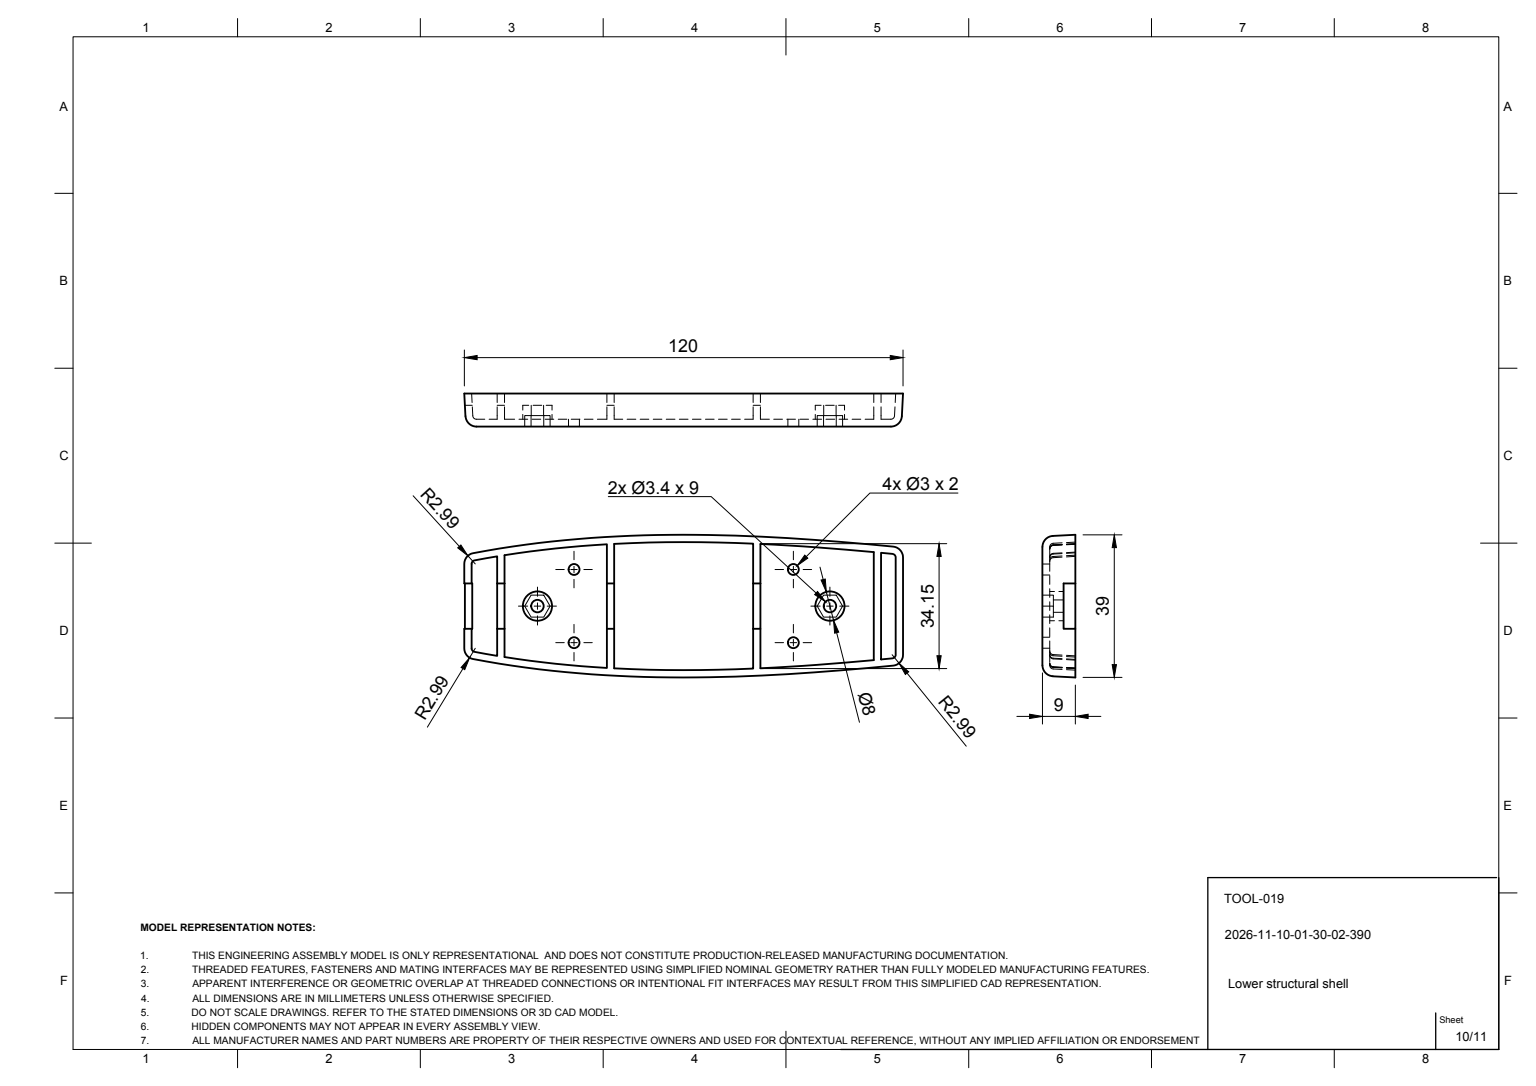
ISO-10303-21;
HEADER;
/* Generated by software containing ST-Developer
 * from STEP Tools, Inc. (www.steptools.com) 
 */

FILE_DESCRIPTION(
/* description */ (''),
/* implementation_level */ '2;1');

FILE_NAME(
/* name */ 'Lower structural shell.step',
/* time_stamp */ '2026-11-10T09:14:46-08:00',
/* author */ (''),
/* organization */ (''),
/* preprocessor_version */ 'ST-DEVELOPER v20.2',
/* originating_system */ 'Autodesk Translation Framework v15.17.0.0',
/* authorisation */ '');

FILE_SCHEMA (('AUTOMOTIVE_DESIGN { 1 0 10303 214 3 1 1 }'));
ENDSEC;

DATA;
#10=MECHANICAL_DESIGN_GEOMETRIC_PRESENTATION_REPRESENTATION('',(#563),#19471);
#84=SPHERICAL_SURFACE('',#7596,0.0999999999999999);
#85=SPHERICAL_SURFACE('',#7599,0.100000000000002);
#86=SPHERICAL_SURFACE('',#7603,0.0999999999999991);
#87=SPHERICAL_SURFACE('',#7607,0.1);
#88=SPHERICAL_SURFACE('',#7612,0.3);
#89=SPHERICAL_SURFACE('',#7616,0.300000000000002);
#90=SPHERICAL_SURFACE('',#7620,0.299999999999999);
#91=SPHERICAL_SURFACE('',#7625,0.3);
#124=B_SPLINE_SURFACE_WITH_KNOTS('',3,3,((#12681,#12682,#12683,#12684),
(#12685,#12686,#12687,#12688),(#12689,#12690,#12691,#12692),(#12693,#12694,
#12695,#12696)),.UNSPECIFIED.,.F.,.F.,.F.,(4,4),(4,4),(0.0627625298587661,
0.3242096015809),(0.0118073085896899,0.685451490706028),.UNSPECIFIED.);
#125=B_SPLINE_SURFACE_WITH_KNOTS('',3,3,((#12701,#12702,#12703,#12704),
(#12705,#12706,#12707,#12708),(#12709,#12710,#12711,#12712),(#12713,#12714,
#12715,#12716)),.UNSPECIFIED.,.F.,.F.,.F.,(4,4),(4,4),(0.0225360950145449,
0.0483865590996774),(0.0125659096559557,0.685650832343257),
 .UNSPECIFIED.);
#126=B_SPLINE_SURFACE_WITH_KNOTS('',3,3,((#12726,#12727,#12728,#12729),
(#12730,#12731,#12732,#12733),(#12734,#12735,#12736,#12737),(#12738,#12739,
#12740,#12741),(#12742,#12743,#12744,#12745)),.UNSPECIFIED.,.F.,.F.,.F.,
(4,1,4),(4,4),(0.,0.571428571428571,1.),(0.74118252158834,3.85438678954986),
 .UNSPECIFIED.);
#127=B_SPLINE_SURFACE_WITH_KNOTS('',3,3,((#12750,#12751,#12752,#12753),
(#12754,#12755,#12756,#12757),(#12758,#12759,#12760,#12761),(#12762,#12763,
#12764,#12765),(#12766,#12767,#12768,#12769)),.UNSPECIFIED.,.F.,.F.,.F.,
(4,1,4),(4,4),(0.,0.571428571428571,1.),(0.270878787657975,0.54981857912664),
 .UNSPECIFIED.);
#128=B_SPLINE_SURFACE_WITH_KNOTS('',3,3,((#12788,#12789,#12790,#12791),
(#12792,#12793,#12794,#12795),(#12796,#12797,#12798,#12799),(#12800,#12801,
#12802,#12803),(#12804,#12805,#12806,#12807)),.UNSPECIFIED.,.F.,.F.,.F.,
(4,1,4),(4,4),(0.,0.571428571428571,1.),(8.03948512627517,11.1526893942367),
 .UNSPECIFIED.);
#129=B_SPLINE_SURFACE_WITH_KNOTS('',3,3,((#12812,#12813,#12814,#12815),
(#12816,#12817,#12818,#12819),(#12820,#12821,#12822,#12823),(#12824,#12825,
#12826,#12827)),.UNSPECIFIED.,.F.,.F.,.F.,(4,4),(4,4),(0.675790398419059,
0.937237470141233),(0.0118073085603101,0.685451490706029),.UNSPECIFIED.);
#130=B_SPLINE_SURFACE_WITH_KNOTS('',3,3,((#12828,#12829,#12830,#12831),
(#12832,#12833,#12834,#12835),(#12836,#12837,#12838,#12839),(#12840,#12841,
#12842,#12843)),.UNSPECIFIED.,.F.,.F.,.F.,(4,4),(4,4),(0.951613440900322,
0.977463904985455),(0.0125659096559558,0.685650832343257),.UNSPECIFIED.);
#131=B_SPLINE_SURFACE_WITH_KNOTS('',3,3,((#12927,#12928,#12929,#12930),
(#12931,#12932,#12933,#12934),(#12935,#12936,#12937,#12938),(#12939,#12940,
#12941,#12942)),.UNSPECIFIED.,.F.,.F.,.F.,(4,4),(4,4),(0.340089900275858,
0.660082688299826),(0.0116294244283504,0.684384408933581),.UNSPECIFIED.);
#132=B_SPLINE_SURFACE_WITH_KNOTS('',3,3,((#12947,#12948,#12949,#12950),
(#12951,#12952,#12953,#12954),(#12955,#12956,#12957,#12958),(#12959,#12960,
#12961,#12962),(#12963,#12964,#12965,#12966)),.UNSPECIFIED.,.F.,.F.,.F.,
(4,1,4),(4,4),(0.,0.571428571428571,1.),(4.04989375377528,7.85140214144331),
 .UNSPECIFIED.);
#133=B_SPLINE_SURFACE_WITH_KNOTS('',3,3,((#12976,#12977,#12978,#12979),
(#12980,#12981,#12982,#12983),(#12984,#12985,#12986,#12987),(#12988,#12989,
#12990,#12991),(#12992,#12993,#12994,#12995)),.UNSPECIFIED.,.F.,.F.,.F.,
(4,1,4),(4,4),(0.,0.571428571428571,1.),(4.0424697743818,7.84397816204974),
 .UNSPECIFIED.);
#134=B_SPLINE_SURFACE_WITH_KNOTS('',3,3,((#13000,#13001,#13002,#13003),
(#13004,#13005,#13006,#13007),(#13008,#13009,#13010,#13011),(#13012,#13013,
#13014,#13015)),.UNSPECIFIED.,.F.,.F.,.F.,(4,4),(4,4),(0.339917311700174,
0.659910099724142),(0.0116294573698948,0.684384408933581),.UNSPECIFIED.);
#135=B_SPLINE_SURFACE_WITH_KNOTS('',3,3,((#13090,#13091,#13092,#13093),
(#13094,#13095,#13096,#13097),(#13098,#13099,#13100,#13101),(#13102,#13103,
#13104,#13105)),.UNSPECIFIED.,.F.,.F.,.F.,(4,4),(4,4),(0.675996615945502,
0.913173856075534),(0.0118505108223707,0.686152089762332),.UNSPECIFIED.);
#136=B_SPLINE_SURFACE_WITH_KNOTS('',3,3,((#13110,#13111,#13112,#13113),
(#13114,#13115,#13116,#13117),(#13118,#13119,#13120,#13121),(#13122,#13123,
#13124,#13125),(#13126,#13127,#13128,#13129)),.UNSPECIFIED.,.F.,.F.,.F.,
(4,1,4),(4,4),(0.,0.571428571428571,1.),(8.0457708503995,10.8690635835914),
 .UNSPECIFIED.);
#137=B_SPLINE_SURFACE_WITH_KNOTS('',3,3,((#13139,#13140,#13141,#13142),
(#13143,#13144,#13145,#13146),(#13147,#13148,#13149,#13150),(#13151,#13152,
#13153,#13154),(#13155,#13156,#13157,#13158)),.UNSPECIFIED.,.F.,.F.,.F.,
(4,1,4),(4,4),(0.,0.571428571428571,1.),(1.02480833223363,3.8481010654256),
 .UNSPECIFIED.);
#138=B_SPLINE_SURFACE_WITH_KNOTS('',3,3,((#13163,#13164,#13165,#13166),
(#13167,#13168,#13169,#13170),(#13171,#13172,#13173,#13174),(#13175,#13176,
#13177,#13178)),.UNSPECIFIED.,.F.,.F.,.F.,(4,4),(4,4),(0.0868261439244655,
0.324003384054498),(0.0118505108223707,0.686152089762332),.UNSPECIFIED.);
#139=B_SPLINE_SURFACE_WITH_KNOTS('',3,3,((#13253,#13254,#13255,#13256),
(#13257,#13258,#13259,#13260),(#13261,#13262,#13263,#13264),(#13265,#13266,
#13267,#13268)),.UNSPECIFIED.,.F.,.F.,.F.,(4,4),(4,4),(0.927751606342899,
0.979699913047832),(0.0130895688562318,0.686930956013783),.UNSPECIFIED.);
#140=B_SPLINE_SURFACE_WITH_KNOTS('',3,3,((#13278,#13279,#13280,#13281),
(#13282,#13283,#13284,#13285),(#13286,#13287,#13288,#13289),(#13290,#13291,
#13292,#13293),(#13294,#13295,#13296,#13297)),.UNSPECIFIED.,.F.,.F.,.F.,
(4,1,4),(4,4),(0.,0.571428571428571,1.),(11.0550486447215,11.6488871259622),
 .UNSPECIFIED.);
#141=B_SPLINE_SURFACE_WITH_KNOTS('',3,3,((#13311,#13312,#13313,#13314),
(#13315,#13316,#13317,#13318),(#13319,#13320,#13321,#13322),(#13323,#13324,
#13325,#13326)),.UNSPECIFIED.,.F.,.F.,.F.,(4,4),(4,4),(0.0203000869521683,
0.0722483936571013),(0.0130895688562318,0.686930956013783),
 .UNSPECIFIED.);
#142=B_SPLINE_SURFACE_WITH_KNOTS('',3,3,((#13336,#13337,#13338,#13339),
(#13340,#13341,#13342,#13343),(#13344,#13345,#13346,#13347),(#13348,#13349,
#13350,#13351),(#13352,#13353,#13354,#13355)),.UNSPECIFIED.,.F.,.F.,.F.,
(4,1,4),(4,4),(0.,0.571428571428571,1.),(0.244984789862841,0.838823271103535),
 .UNSPECIFIED.);
#143=B_SPLINE_SURFACE_WITH_KNOTS('',3,3,((#13369,#13370,#13371,#13372),
(#13373,#13374,#13375,#13376),(#13377,#13378,#13379,#13380),(#13381,#13382,
#13383,#13384),(#13385,#13386,#13387,#13388)),.UNSPECIFIED.,.F.,.F.,.F.,
(4,1,4),(4,4),(0.,0.5,1.),(0.0108921325678979,0.619909717328002),
 .UNSPECIFIED.);
#144=B_SPLINE_SURFACE_WITH_KNOTS('',3,3,((#13395,#13396,#13397,#13398),
(#13399,#13400,#13401,#13402),(#13403,#13404,#13405,#13406),(#13407,#13408,
#13409,#13410),(#13411,#13412,#13413,#13414)),.UNSPECIFIED.,.F.,.F.,.F.,
(4,1,4),(4,4),(0.,0.571428571428571,1.),(0.00967450486392679,0.618764321025346),
 .UNSPECIFIED.);
#145=B_SPLINE_SURFACE_WITH_KNOTS('',3,3,((#13419,#13420,#13421,#13422),
(#13423,#13424,#13425,#13426),(#13427,#13428,#13429,#13430),(#13431,#13432,
#13433,#13434),(#13435,#13436,#13437,#13438)),.UNSPECIFIED.,.F.,.F.,.F.,
(4,1,4),(4,4),(0.,0.571428571428571,1.),(0.0097274579809394,0.618764321025346),
 .UNSPECIFIED.);
#146=B_SPLINE_SURFACE_WITH_KNOTS('',3,3,((#13443,#13444,#13445,#13446),
(#13447,#13448,#13449,#13450),(#13451,#13452,#13453,#13454),(#13455,#13456,
#13457,#13458),(#13459,#13460,#13461,#13462)),.UNSPECIFIED.,.F.,.F.,.F.,
(4,1,4),(4,4),(0.,0.571428571428571,1.),(11.3440533366984,11.6229931281671),
 .UNSPECIFIED.);
#147=B_SPLINE_SURFACE_WITH_KNOTS('',3,3,((#13463,#13464,#13465,#13466),
(#13467,#13468,#13469,#13470),(#13471,#13472,#13473,#13474),(#13475,#13476,
#13477,#13478),(#13479,#13480,#13481,#13482)),.UNSPECIFIED.,.F.,.F.,.F.,
(4,1,4),(4,4),(0.,0.5,1.),(0.0108402259132964,0.619909717328002),
 .UNSPECIFIED.);
#148=B_SPLINE_SURFACE_WITH_KNOTS('',3,3,((#13508,#13509,#13510,#13511),
(#13512,#13513,#13514,#13515),(#13516,#13517,#13518,#13519),(#13520,#13521,
#13522,#13523),(#13524,#13525,#13526,#13527)),.UNSPECIFIED.,.F.,.F.,.F.,
(4,1,4),(4,4),(0.,0.571428571428571,1.),(-0.00387706229521417,0.619909717328002),
 .UNSPECIFIED.);
#149=B_SPLINE_SURFACE_WITH_KNOTS('',3,3,((#13546,#13547,#13548,#13549,#13550,
#13551),(#13552,#13553,#13554,#13555,#13556,#13557),(#13558,#13559,#13560,
#13561,#13562,#13563),(#13564,#13565,#13566,#13567,#13568,#13569),(#13570,
#13571,#13572,#13573,#13574,#13575)),.UNSPECIFIED.,.F.,.F.,.F.,(4,1,4),
(4,1,1,4),(0.,0.571428571428571,1.),(0.270878787657975,5.14716807550265,
8.39802760073243,11.6488871259622),.UNSPECIFIED.);
#150=B_SPLINE_SURFACE_WITH_KNOTS('',3,3,((#13588,#13589,#13590,#13591),
(#13592,#13593,#13594,#13595),(#13596,#13597,#13598,#13599),(#13600,#13601,
#13602,#13603),(#13604,#13605,#13606,#13607)),.UNSPECIFIED.,.F.,.F.,.F.,
(4,1,4),(4,4),(0.,0.571428571428571,1.),(-0.00522825793187074,0.618764321025346),
 .UNSPECIFIED.);
#151=B_SPLINE_SURFACE_WITH_KNOTS('',3,3,((#13616,#13617,#13618,#13619),
(#13620,#13621,#13622,#13623),(#13624,#13625,#13626,#13627),(#13628,#13629,
#13630,#13631),(#13632,#13633,#13634,#13635)),.UNSPECIFIED.,.F.,.F.,.F.,
(4,1,4),(4,4),(0.,0.571428571428571,1.),(-0.00506942997988007,0.618764321025346),
 .UNSPECIFIED.);
#152=B_SPLINE_SURFACE_WITH_KNOTS('',3,3,((#13644,#13645,#13646,#13647,#13648),
(#13649,#13650,#13651,#13652,#13653),(#13654,#13655,#13656,#13657,#13658),
(#13659,#13660,#13661,#13662,#13663),(#13664,#13665,#13666,#13667,#13668)),
 .UNSPECIFIED.,.F.,.F.,.F.,(4,1,4),(4,1,4),(0.,0.571428571428571,1.),(0.244984789862841,
5.12127407770751,11.6229931281671),.UNSPECIFIED.);
#153=B_SPLINE_SURFACE_WITH_KNOTS('',3,3,((#13679,#13680,#13681,#13682),
(#13683,#13684,#13685,#13686),(#13687,#13688,#13689,#13690),(#13691,#13692,
#13693,#13694),(#13695,#13696,#13697,#13698)),.UNSPECIFIED.,.F.,.F.,.F.,
(4,1,4),(4,4),(0.,0.571428571428571,1.),(-0.00403278922781227,0.619909717328002),
 .UNSPECIFIED.);
#154=B_SPLINE_SURFACE_WITH_KNOTS('',3,3,((#13707,#13708,#13709,#13710),
(#13711,#13712,#13713,#13714),(#13715,#13716,#13717,#13718),(#13719,#13720,
#13721,#13722)),.UNSPECIFIED.,.F.,.F.,.F.,(4,4),(4,4),(0.0225340877622934,
0.979701609653785),(0.,0.686930956013783),.UNSPECIFIED.);
#155=B_SPLINE_SURFACE_WITH_KNOTS('',3,3,((#13725,#13726,#13727,#13728),
(#13729,#13730,#13731,#13732),(#13733,#13734,#13735,#13736),(#13737,#13738,
#13739,#13740)),.UNSPECIFIED.,.F.,.F.,.F.,(4,4),(4,4),(0.0202983903462145,
0.977465912237707),(0.,0.686930956013783),.UNSPECIFIED.);
#264=B_SPLINE_CURVE_WITH_KNOTS('',3,(#11953,#11954,#11955,#11956,#11957,
#11958),.UNSPECIFIED.,.F.,.F.,(4,2,4),(-0.607240122656937,-0.303691721894415,
-0.000634514333697656),.UNSPECIFIED.);
#265=B_SPLINE_CURVE_WITH_KNOTS('',3,(#11960,#11961,#11962,#11963,#11964,
#11965,#11966,#11967,#11968,#11969,#11970,#11971,#11972,#11973,#11974,#11975,
#11976,#11977,#11978,#11979,#11980,#11981,#11982,#11983,#11984,#11985,#11986,
#11987),.UNSPECIFIED.,.F.,.F.,(4,3,3,3,3,3,3,3,3,4),(-0.152223584381152,
-0.128403685910756,-0.115058138924018,-0.0911105876986024,-0.0779275105489685,
-0.0651650823668383,-0.0413494676927402,-0.0389105926748606,-0.0151313403168948,
0.),.UNSPECIFIED.);
#266=B_SPLINE_CURVE_WITH_KNOTS('',3,(#11991,#11992,#11993,#11994,#11995,
#11996,#11997,#11998,#11999,#12000,#12001,#12002,#12003,#12004,#12005,#12006,
#12007,#12008,#12009,#12010,#12011,#12012,#12013,#12014,#12015,#12016,#12017,
#12018),.UNSPECIFIED.,.F.,.F.,(4,3,3,3,3,3,3,3,3,4),(-0.152249917238265,
-0.128484865669312,-0.115494642307313,-0.0916985948709881,-0.0870953287403626,
-0.0787006597758974,-0.0547717013112817,-0.0393956522318865,-0.0155460991587222,
0.),.UNSPECIFIED.);
#267=B_SPLINE_CURVE_WITH_KNOTS('',3,(#12019,#12020,#12021,#12022,#12023,
#12024),.UNSPECIFIED.,.F.,.F.,(4,2,4),(-0.606785315485727,-0.30369188913634,
-0.000179692314978108),.UNSPECIFIED.);
#268=B_SPLINE_CURVE_WITH_KNOTS('',3,(#12029,#12030,#12031,#12032,#12033,
#12034),.UNSPECIFIED.,.F.,.F.,(4,2,4),(-0.606332812995025,-0.303737653350621,
-0.000161665236032726),.UNSPECIFIED.);
#269=B_SPLINE_CURVE_WITH_KNOTS('',3,(#12036,#12037,#12038,#12039,#12040,
#12041,#12042,#12043,#12044,#12045,#12046,#12047,#12048,#12049,#12050,#12051,
#12052,#12053,#12054,#12055,#12056,#12057,#12058,#12059,#12060,#12061,#12062,
#12063),.UNSPECIFIED.,.F.,.F.,(4,3,3,3,3,3,3,3,3,4),(-0.152301160038588,
-0.128555435257278,-0.115184785848022,-0.0912639339035621,-0.0780773216554274,
-0.065267350293706,-0.0414723266145325,-0.0390252168402571,-0.0152374671294611,
0.),.UNSPECIFIED.);
#270=B_SPLINE_CURVE_WITH_KNOTS('',3,(#12067,#12068,#12069,#12070,#12071,
#12072,#12073,#12074,#12075,#12076,#12077,#12078,#12079,#12080,#12081,#12082,
#12083,#12084,#12085,#12086,#12087,#12088,#12089,#12090,#12091,#12092,#12093,
#12094),.UNSPECIFIED.,.F.,.F.,(4,3,3,3,3,3,3,3,3,4),(-0.152307894271445,
-0.128535938708366,-0.115295945509717,-0.0915234088298753,-0.0870575315710991,
-0.0782740392368046,-0.0543664511067997,-0.0391484926712317,-0.0153774171089249,
0.),.UNSPECIFIED.);
#271=B_SPLINE_CURVE_WITH_KNOTS('',3,(#12096,#12097,#12098,#12099,#12100,
#12101),.UNSPECIFIED.,.F.,.F.,(4,2,4),(-0.607315067615316,-0.303737782617996,
-0.00114390098251854),.UNSPECIFIED.);
#272=B_SPLINE_CURVE_WITH_KNOTS('',3,(#12107,#12108,#12109,#12110,#12111,
#12112),.UNSPECIFIED.,.F.,.F.,(4,2,4),(-0.606335618682527,-0.303964064424246,
-0.000163142902895597),.UNSPECIFIED.);
#273=B_SPLINE_CURVE_WITH_KNOTS('',3,(#12114,#12115,#12116,#12117,#12118,
#12119,#12120,#12121,#12122,#12123,#12124,#12125,#12126,#12127,#12128,#12129,
#12130,#12131,#12132,#12133,#12134,#12135,#12136,#12137,#12138,#12139,#12140,
#12141),.UNSPECIFIED.,.F.,.F.,(4,3,3,3,3,3,3,3,3,4),(-0.152324888062519,
-0.128571266282871,-0.115187819092559,-0.0912644922975459,-0.0780623053857969,
-0.0652705430018984,-0.0414736125245103,-0.0390138150290758,-0.015226502089553,
0.),.UNSPECIFIED.);
#274=B_SPLINE_CURVE_WITH_KNOTS('',3,(#12145,#12146,#12147,#12148,#12149,
#12150,#12151,#12152,#12153,#12154,#12155,#12156,#12157,#12158,#12159,#12160,
#12161,#12162,#12163,#12164,#12165,#12166,#12167,#12168,#12169,#12170,#12171,
#12172),.UNSPECIFIED.,.F.,.F.,(4,3,3,3,3,3,3,3,3,4),(-0.152333600285603,
-0.128561769460285,-0.115331525958272,-0.0915566852459163,-0.0870792380259527,
-0.0783165909319309,-0.0544069520497563,-0.0391732033593778,-0.0153939862842036,
0.),.UNSPECIFIED.);
#275=B_SPLINE_CURVE_WITH_KNOTS('',3,(#12174,#12175,#12176,#12177,#12178,
#12179),.UNSPECIFIED.,.F.,.F.,(4,2,4),(-0.607765665607205,-0.303964210965506,
-0.00159316434717749),.UNSPECIFIED.);
#276=B_SPLINE_CURVE_WITH_KNOTS('',3,(#12185,#12186,#12187,#12188,#12189,
#12190),.UNSPECIFIED.,.F.,.F.,(4,2,4),(-0.608113833554089,-0.304405910662044,
-0.00120843896277512),.UNSPECIFIED.);
#277=B_SPLINE_CURVE_WITH_KNOTS('',3,(#12192,#12193,#12194,#12195,#12196,
#12197,#12198,#12199,#12200,#12201,#12202,#12203,#12204,#12205,#12206,#12207,
#12208,#12209,#12210,#12211,#12212,#12213,#12214,#12215,#12216,#12217,#12218,
#12219),.UNSPECIFIED.,.F.,.F.,(4,3,3,3,3,3,3,3,3,4),(-0.152638346832965,
-0.128647829044501,-0.117000727359648,-0.0929750760194364,-0.0775532335837778,
-0.065166230851578,-0.0413072760700971,-0.0386249916896363,-0.0148681833632798,
0.),.UNSPECIFIED.);
#278=B_SPLINE_CURVE_WITH_KNOTS('',3,(#12223,#12224,#12225,#12226,#12227,
#12228,#12229,#12230,#12231,#12232,#12233,#12234,#12235,#12236,#12237,#12238,
#12239,#12240,#12241,#12242,#12243,#12244,#12245,#12246,#12247,#12248,#12249,
#12250),.UNSPECIFIED.,.F.,.F.,(4,3,3,3,3,3,3,3,3,4),(-0.152712908768378,
-0.128963682254188,-0.116304008925778,-0.092453135123643,-0.0875380734791113,
-0.0797852913889514,-0.0558105568475602,-0.0400274901149945,-0.0159798645019078,
0.),.UNSPECIFIED.);
#279=B_SPLINE_CURVE_WITH_KNOTS('',3,(#12252,#12253,#12254,#12255,#12256,
#12257),.UNSPECIFIED.,.F.,.F.,(4,2,4),(-0.607607610897069,-0.304406883675693,
-0.000702187548907163),.UNSPECIFIED.);
#280=B_SPLINE_CURVE_WITH_KNOTS('',3,(#12263,#12264,#12265,#12266),
 .UNSPECIFIED.,.F.,.F.,(4,4),(0.0130288733793136,0.619909717328002),
 .UNSPECIFIED.);
#281=B_SPLINE_CURVE_WITH_KNOTS('',3,(#12270,#12271,#12272,#12273),
 .UNSPECIFIED.,.F.,.F.,(4,4),(-0.619909717328002,-0.0130288733793137),
 .UNSPECIFIED.);
#282=B_SPLINE_CURVE_WITH_KNOTS('',3,(#12276,#12277,#12278,#12279,#12280,
#12281,#12282),.UNSPECIFIED.,.F.,.F.,(4,3,4),(7.87274532319472,10.4298004347969,
10.9780233963721),.UNSPECIFIED.);
#283=B_SPLINE_CURVE_WITH_KNOTS('',3,(#12283,#12284,#12285,#12286,#12287,
#12288,#12289),.UNSPECIFIED.,.F.,.F.,(4,3,4),(0.511752108249611,2.84807862798167,
3.61537599721027),.UNSPECIFIED.);
#284=B_SPLINE_CURVE_WITH_KNOTS('',3,(#12292,#12293,#12294,#12295,#12296,
#12297,#12298),.UNSPECIFIED.,.F.,.F.,(4,3,4),(3.81523717927831,5.72635044542746,
7.61820606472736),.UNSPECIFIED.);
#285=B_SPLINE_CURVE_WITH_KNOTS('',3,(#12301,#12302,#12303,#12304),
 .UNSPECIFIED.,.F.,.F.,(4,4),(7.8195516254834,10.6519234170402),
 .UNSPECIFIED.);
#286=B_SPLINE_CURVE_WITH_KNOTS('',3,(#12308,#12309,#12310,#12311),
 .UNSPECIFIED.,.F.,.F.,(4,4),(10.8550709503701,11.4839159448819),
 .UNSPECIFIED.);
#287=B_SPLINE_CURVE_WITH_KNOTS('',3,(#12312,#12313,#12314,#12315,#12316,
#12317,#12318,#12319,#12320,#12321,#12322,#12323,#12324,#12325,#12326,#12327,
#12328,#12329,#12330,#12331,#12332,#12333,#12334,#12335,#12336,#12337,#12338,
#12339),.UNSPECIFIED.,.F.,.F.,(4,3,3,3,3,3,3,3,3,4),(0.,0.023800266251022,
0.0390470051780055,0.062864594207143,0.0692752090304052,0.0780196763370091,
0.101808338076191,0.108235461704482,0.131970324379069,0.138468980573541),
 .UNSPECIFIED.);
#288=B_SPLINE_CURVE_WITH_KNOTS('',3,(#12343,#12344,#12345,#12346,#12347,
#12348,#12349,#12350,#12351,#12352,#12353,#12354,#12355,#12356,#12357,#12358,
#12359,#12360,#12361,#12362,#12363,#12364,#12365,#12366,#12367,#12368,#12369,
#12370,#12371,#12372,#12373),.UNSPECIFIED.,.F.,.F.,(4,3,3,3,3,3,3,3,3,3,
4),(0.,0.0536158767337707,0.107707970980176,0.117140678528723,0.171373940961503,
0.178118425384842,0.234058785038521,0.2884659822146,0.324708667187819,0.378759781373182,
0.415412568437851),.UNSPECIFIED.);
#289=B_SPLINE_CURVE_WITH_KNOTS('',3,(#12375,#12376,#12377,#12378),
 .UNSPECIFIED.,.F.,.F.,(4,4),(0.0202983903462145,0.977465912237707),
 .UNSPECIFIED.);
#290=B_SPLINE_CURVE_WITH_KNOTS('',3,(#12380,#12381,#12382,#12383,#12384,
#12385,#12386,#12387,#12388,#12389,#12390,#12391,#12392,#12393,#12394,#12395,
#12396,#12397,#12398,#12399,#12400,#12401,#12402,#12403,#12404,#12405,#12406,
#12407,#12408,#12409,#12410),.UNSPECIFIED.,.F.,.F.,(4,3,3,3,3,3,3,3,3,3,
4),(0.,0.053547205187505,0.107728964525782,0.117299670245694,0.171524652009909,
0.189842726242433,0.234296321023441,0.288773621215207,0.338477936388461,
0.392564001789548,0.442713223041249),.UNSPECIFIED.);
#291=B_SPLINE_CURVE_WITH_KNOTS('',3,(#12414,#12415,#12416,#12417,#12418,
#12419,#12420,#12421,#12422,#12423,#12424,#12425,#12426,#12427,#12428,#12429,
#12430,#12431,#12432,#12433,#12434,#12435,#12436,#12437,#12438,#12439,#12440,
#12441,#12442,#12443,#12444),.UNSPECIFIED.,.F.,.F.,(4,3,3,3,3,3,3,3,3,3,
4),(0.,0.0535312152416108,0.107707123412492,0.117215931328448,0.171445047002381,
0.189808362521926,0.234165405003858,0.288639615809812,0.338404447092272,
0.392504428396833,0.442708851597914),.UNSPECIFIED.);
#292=B_SPLINE_CURVE_WITH_KNOTS('',3,(#12446,#12447,#12448,#12449),
 .UNSPECIFIED.,.F.,.F.,(4,4),(0.0225340877622936,0.979701609653785),
 .UNSPECIFIED.);
#293=B_SPLINE_CURVE_WITH_KNOTS('',3,(#12451,#12452,#12453,#12454,#12455,
#12456,#12457,#12458,#12459,#12460,#12461,#12462,#12463,#12464,#12465,#12466,
#12467,#12468,#12469,#12470,#12471,#12472,#12473,#12474,#12475,#12476,#12477,
#12478,#12479,#12480,#12481),.UNSPECIFIED.,.F.,.F.,(4,3,3,3,3,3,3,3,3,3,
4),(0.,0.0536458552170769,0.107744721567334,0.117297895480617,0.171522683869793,
0.178177673384308,0.23429412186666,0.288702228477357,0.324838815929715,
0.378862861687027,0.415420074045746),.UNSPECIFIED.);
#294=B_SPLINE_CURVE_WITH_KNOTS('',3,(#12484,#12485,#12486,#12487,#12488,
#12489,#12490,#12491,#12492,#12493,#12494,#12495,#12496,#12497,#12498,#12499,
#12500,#12501,#12502,#12503,#12504,#12505,#12506,#12507,#12508,#12509,#12510,
#12511),.UNSPECIFIED.,.F.,.F.,(4,3,3,3,3,3,3,3,3,4),(0.,0.0238098951475563,
0.0390995920428052,0.0629117710415135,0.0692953339558167,0.0780985718814299,
0.101889748471939,0.108278926258091,0.132003149848588,0.138471484390145),
 .UNSPECIFIED.);
#295=B_SPLINE_CURVE_WITH_KNOTS('',3,(#12513,#12514,#12515,#12516),
 .UNSPECIFIED.,.F.,.F.,(4,4),(2.05597917304345E-5,0.629200412657851),
 .UNSPECIFIED.);
#296=B_SPLINE_CURVE_WITH_KNOTS('',3,(#12519,#12520,#12521,#12522),
 .UNSPECIFIED.,.F.,.F.,(4,4),(0.832456091119126,3.6663340257767),
 .UNSPECIFIED.);
#297=B_SPLINE_CURVE_WITH_KNOTS('',3,(#12525,#12526,#12527,#12528,#12529,
#12530,#12531),.UNSPECIFIED.,.F.,.F.,(4,3,4),(3.86778652923942,5.76006783397632,
7.67277763234621),.UNSPECIFIED.);
#298=B_SPLINE_CURVE_WITH_KNOTS('',3,(#12535,#12536,#12537,#12538),
 .UNSPECIFIED.,.F.,.F.,(4,4),(11.1789026308149,11.490024089745),
 .UNSPECIFIED.);
#299=B_SPLINE_CURVE_WITH_KNOTS('',3,(#12540,#12541,#12542,#12543,#12544,
#12545,#12546,#12547,#12548,#12549,#12550,#12551,#12552,#12553,#12554,#12555,
#12556,#12557,#12558,#12559,#12560,#12561,#12562,#12563,#12564),
 .UNSPECIFIED.,.F.,.F.,(4,3,3,3,3,3,3,3,4),(0.,0.0238050540413609,0.0390723036702896,
0.0632692088215501,0.0780555758269344,0.101951849921082,0.112801451778717,
0.136536488207902,0.147568670144067),.UNSPECIFIED.);
#300=B_SPLINE_CURVE_WITH_KNOTS('',3,(#12568,#12569,#12570,#12571,#12572,
#12573,#12574,#12575,#12576,#12577,#12578,#12579,#12580,#12581,#12582,#12583,
#12584,#12585,#12586,#12587,#12588,#12589,#12590,#12591,#12592),
 .UNSPECIFIED.,.F.,.F.,(4,3,3,3,3,3,3,3,4),(0.,0.0238098889950854,0.0391003179068551,
0.0632803937136523,0.0780994777107358,0.101997157448698,0.112825962756833,
0.136555142506291,0.147570127973408),.UNSPECIFIED.);
#301=B_SPLINE_CURVE_WITH_KNOTS('',3,(#12594,#12595,#12596,#12597),
 .UNSPECIFIED.,.F.,.F.,(4,4),(2.41556456535008E-5,0.310979882704647),
 .UNSPECIFIED.);
#302=B_SPLINE_CURVE_WITH_KNOTS('',3,(#12609,#12610,#12611,#12612,#12613,
#12614),.UNSPECIFIED.,.F.,.F.,(4,2,4),(-0.606744425054929,-0.30369469419025,
-0.000104868936493974),.UNSPECIFIED.);
#303=B_SPLINE_CURVE_WITH_KNOTS('',3,(#12616,#12617,#12618,#12619,#12620,
#12621),.UNSPECIFIED.,.F.,.F.,(4,2,4),(-0.60732337425873,-0.303694522808999,
-0.000683832228057069),.UNSPECIFIED.);
#304=B_SPLINE_CURVE_WITH_KNOTS('',3,(#12623,#12624,#12625,#12626,#12627,
#12628,#12629,#12630,#12631,#12632,#12633,#12634,#12635,#12636,#12637,#12638,
#12639,#12640,#12641,#12642,#12643,#12644,#12645,#12646,#12647,#12648,#12649,
#12650),.UNSPECIFIED.,.F.,.F.,(4,3,3,3,3,3,3,3,3,4),(-0.152213081758773,
-0.128388856548194,-0.115047734630008,-0.0910986092737131,-0.0779187269986961,
-0.0651565114518209,-0.0413397067626705,-0.0389038209724845,-0.0151251319644201,
0.),.UNSPECIFIED.);
#305=B_SPLINE_CURVE_WITH_KNOTS('',3,(#12653,#12654,#12655,#12656,#12657,
#12658,#12659,#12660,#12661,#12662,#12663,#12664,#12665,#12666,#12667,#12668,
#12669,#12670,#12671,#12672,#12673,#12674,#12675,#12676,#12677,#12678,#12679,
#12680),.UNSPECIFIED.,.F.,.F.,(4,3,3,3,3,3,3,3,3,4),(-0.152240567100014,
-0.128476012965191,-0.115503482174674,-0.0917060839439778,-0.0870941983819305,
-0.0787260045726768,-0.0547958477503903,-0.0394103419198022,-0.0155561788900784,
0.),.UNSPECIFIED.);
#306=B_SPLINE_CURVE_WITH_KNOTS('',3,(#12697,#12698,#12699,#12700),
 .UNSPECIFIED.,.F.,.F.,(4,4),(-3.85438678954986,-0.750511952447855),
 .UNSPECIFIED.);
#307=B_SPLINE_CURVE_WITH_KNOTS('',3,(#12718,#12719,#12720,#12721),
 .UNSPECIFIED.,.F.,.F.,(4,4),(-0.54981857912664,-0.270878787657975),
 .UNSPECIFIED.);
#308=B_SPLINE_CURVE_WITH_KNOTS('',3,(#12722,#12723,#12724,#12725),
 .UNSPECIFIED.,.F.,.F.,(4,4),(-0.618764321025346,-0.0114172178585034),
 .UNSPECIFIED.);
#309=B_SPLINE_CURVE_WITH_KNOTS('',3,(#12746,#12747,#12748,#12749),
 .UNSPECIFIED.,.F.,.F.,(4,4),(0.74118252158834,3.84969085360113),
 .UNSPECIFIED.);
#310=B_SPLINE_CURVE_WITH_KNOTS('',3,(#12771,#12772,#12773,#12774),
 .UNSPECIFIED.,.F.,.F.,(4,4),(0.270878787657975,0.540284107299618),
 .UNSPECIFIED.);
#311=B_SPLINE_CURVE_WITH_KNOTS('',3,(#12777,#12778,#12779,#12780),
 .UNSPECIFIED.,.F.,.F.,(4,4),(8.04418106222393,11.1526893942367),
 .UNSPECIFIED.);
#312=B_SPLINE_CURVE_WITH_KNOTS('',3,(#12783,#12784,#12785,#12786),
 .UNSPECIFIED.,.F.,.F.,(4,4),(11.3535878085254,11.6229931281671),
 .UNSPECIFIED.);
#313=B_SPLINE_CURVE_WITH_KNOTS('',3,(#12808,#12809,#12810,#12811),
 .UNSPECIFIED.,.F.,.F.,(4,4),(-11.1433599633772,-8.03948512627517),
 .UNSPECIFIED.);
#314=B_SPLINE_CURVE_WITH_KNOTS('',3,(#12845,#12846,#12847,#12848),
 .UNSPECIFIED.,.F.,.F.,(4,4),(0.0114172178585033,0.618764321025346),
 .UNSPECIFIED.);
#315=B_SPLINE_CURVE_WITH_KNOTS('',3,(#12849,#12850,#12851,#12852),
 .UNSPECIFIED.,.F.,.F.,(4,4),(-11.6229931281671,-11.3440533366984),
 .UNSPECIFIED.);
#316=B_SPLINE_CURVE_WITH_KNOTS('',3,(#12855,#12856,#12857,#12858,#12859,
#12860),.UNSPECIFIED.,.F.,.F.,(4,2,4),(-0.606286853269513,-0.303735636734938,
-0.000134370544016882),.UNSPECIFIED.);
#317=B_SPLINE_CURVE_WITH_KNOTS('',3,(#12862,#12863,#12864,#12865,#12866,
#12867,#12868,#12869,#12870,#12871,#12872,#12873,#12874,#12875,#12876,#12877,
#12878,#12879,#12880,#12881,#12882,#12883,#12884,#12885,#12886,#12887,#12888,
#12889),.UNSPECIFIED.,.F.,.F.,(4,3,3,3,3,3,3,3,3,4),(-0.152301724526365,
-0.128559761662057,-0.115189905045126,-0.0912708316251271,-0.0780855696141105,
-0.0652713768517459,-0.0414777101816728,-0.0390314967756457,-0.015242903619151,
0.),.UNSPECIFIED.);
#318=B_SPLINE_CURVE_WITH_KNOTS('',3,(#12893,#12894,#12895,#12896,#12897,
#12898,#12899,#12900,#12901,#12902,#12903,#12904,#12905,#12906,#12907,#12908,
#12909,#12910,#12911,#12912,#12913,#12914,#12915,#12916,#12917,#12918,#12919,
#12920),.UNSPECIFIED.,.F.,.F.,(4,3,3,3,3,3,3,3,3,4),(-0.1523073815286,-0.1285346644938,
-0.115283264026726,-0.0915123087981378,-0.0870533687950649,-0.0782507800682277,
-0.0543447803816484,-0.0391350231834537,-0.0153679399182895,0.),
 .UNSPECIFIED.);
#319=B_SPLINE_CURVE_WITH_KNOTS('',3,(#12921,#12922,#12923,#12924,#12925,
#12926),.UNSPECIFIED.,.F.,.F.,(4,2,4),(-0.607338074051965,-0.303735662161239,
-0.00118557149519966),.UNSPECIFIED.);
#320=B_SPLINE_CURVE_WITH_KNOTS('',3,(#12943,#12944,#12945,#12946),
 .UNSPECIFIED.,.F.,.F.,(4,4),(-7.8460657686783,-4.05419673417835),
 .UNSPECIFIED.);
#321=B_SPLINE_CURVE_WITH_KNOTS('',3,(#12967,#12968,#12969,#12970),
 .UNSPECIFIED.,.F.,.F.,(4,4),(4.04989375377528,7.85140214144331),
 .UNSPECIFIED.);
#322=B_SPLINE_CURVE_WITH_KNOTS('',3,(#12972,#12973,#12974,#12975),
 .UNSPECIFIED.,.F.,.F.,(4,4),(4.0424697743818,7.84397816204974),
 .UNSPECIFIED.);
#323=B_SPLINE_CURVE_WITH_KNOTS('',3,(#12996,#12997,#12998,#12999),
 .UNSPECIFIED.,.F.,.F.,(4,4),(-7.83967518164668,-4.0478061471468),
 .UNSPECIFIED.);
#324=B_SPLINE_CURVE_WITH_KNOTS('',3,(#13018,#13019,#13020,#13021,#13022,
#13023),.UNSPECIFIED.,.F.,.F.,(4,2,4),(-0.606398914035431,-0.303967092551845,
-0.000200694235479137),.UNSPECIFIED.);
#325=B_SPLINE_CURVE_WITH_KNOTS('',3,(#13025,#13026,#13027,#13028,#13029,
#13030,#13031,#13032,#13033,#13034,#13035,#13036,#13037,#13038,#13039,#13040,
#13041,#13042,#13043,#13044,#13045,#13046,#13047,#13048,#13049,#13050,#13051,
#13052),.UNSPECIFIED.,.F.,.F.,(4,3,3,3,3,3,3,3,3,4),(-0.15233244131821,
-0.128569871170003,-0.115181988990177,-0.0912564475476021,-0.0780459432968613,
-0.0652662335163151,-0.0414674738832469,-0.0390013640446512,-0.0152139229936509,
0.),.UNSPECIFIED.);
#326=B_SPLINE_CURVE_WITH_KNOTS('',3,(#13056,#13057,#13058,#13059,#13060,
#13061,#13062,#13063,#13064,#13065,#13066,#13067,#13068,#13069,#13070,#13071,
#13072,#13073,#13074,#13075,#13076,#13077,#13078,#13079,#13080,#13081,#13082,
#13083),.UNSPECIFIED.,.F.,.F.,(4,3,3,3,3,3,3,3,3,4),(-0.152343297533924,
-0.128571042154168,-0.115361098257144,-0.0915841820623439,-0.0870924557961151,
-0.0783628838319633,-0.0544516462338148,-0.0392000432438046,-0.0154115240971992,
0.),.UNSPECIFIED.);
#327=B_SPLINE_CURVE_WITH_KNOTS('',3,(#13084,#13085,#13086,#13087,#13088,
#13089),.UNSPECIFIED.,.F.,.F.,(4,2,4),(-0.607734321217702,-0.303967174049374,
-0.00153607519677973),.UNSPECIFIED.);
#328=B_SPLINE_CURVE_WITH_KNOTS('',3,(#13106,#13107,#13108,#13109),
 .UNSPECIFIED.,.F.,.F.,(4,4),(-10.8531956503852,-8.0457708503995),
 .UNSPECIFIED.);
#329=B_SPLINE_CURVE_WITH_KNOTS('',3,(#13130,#13131,#13132,#13133),
 .UNSPECIFIED.,.F.,.F.,(4,4),(8.05172912332209,10.8690635835914),
 .UNSPECIFIED.);
#330=B_SPLINE_CURVE_WITH_KNOTS('',3,(#13135,#13136,#13137,#13138),
 .UNSPECIFIED.,.F.,.F.,(4,4),(1.02480833223363,3.84214279250303),
 .UNSPECIFIED.);
#331=B_SPLINE_CURVE_WITH_KNOTS('',3,(#13159,#13160,#13161,#13162),
 .UNSPECIFIED.,.F.,.F.,(4,4),(-3.8481010654256,-1.04067626543981),
 .UNSPECIFIED.);
#332=B_SPLINE_CURVE_WITH_KNOTS('',3,(#13181,#13182,#13183,#13184,#13185,
#13186),.UNSPECIFIED.,.F.,.F.,(4,2,4),(-0.608301643694891,-0.304416323412316,
-0.0013178649037765),.UNSPECIFIED.);
#333=B_SPLINE_CURVE_WITH_KNOTS('',3,(#13188,#13189,#13190,#13191,#13192,
#13193,#13194,#13195,#13196,#13197,#13198,#13199,#13200,#13201,#13202,#13203,
#13204,#13205,#13206,#13207,#13208,#13209,#13210,#13211,#13212,#13213,#13214,
#13215),.UNSPECIFIED.,.F.,.F.,(4,3,3,3,3,3,3,3,3,4),(-0.152679905805259,
-0.128657903528546,-0.116982385578132,-0.0929502017086943,-0.0774957796939621,
-0.0651567901405441,-0.0412920018136918,-0.0385809476656748,-0.0148252868187304,
0.),.UNSPECIFIED.);
#334=B_SPLINE_CURVE_WITH_KNOTS('',3,(#13219,#13220,#13221,#13222,#13223,
#13224,#13225,#13226,#13227,#13228,#13229,#13230,#13231,#13232,#13233,#13234,
#13235,#13236,#13237,#13238,#13239,#13240,#13241,#13242,#13243,#13244,#13245,
#13246),.UNSPECIFIED.,.F.,.F.,(4,3,3,3,3,3,3,3,3,4),(-0.152762160496458,
-0.129013039804674,-0.116418683706179,-0.0925605502531877,-0.0875939536119484,
-0.0799546107253736,-0.055976748465099,-0.0401263304884301,-0.0160466564276224,
0.),.UNSPECIFIED.);
#335=B_SPLINE_CURVE_WITH_KNOTS('',3,(#13247,#13248,#13249,#13250,#13251,
#13252),.UNSPECIFIED.,.F.,.F.,(4,2,4),(-0.607519387555057,-0.304417308507995,
-0.000535579674449116),.UNSPECIFIED.);
#336=B_SPLINE_CURVE_WITH_KNOTS('',3,(#13270,#13271,#13272,#13273),
 .UNSPECIFIED.,.F.,.F.,(4,4),(0.012184405392802,0.619909717328002),
 .UNSPECIFIED.);
#337=B_SPLINE_CURVE_WITH_KNOTS('',3,(#13274,#13275,#13276,#13277),
 .UNSPECIFIED.,.F.,.F.,(4,4),(-11.6488871259622,-11.0550486447215),
 .UNSPECIFIED.);
#338=B_SPLINE_CURVE_WITH_KNOTS('',3,(#13300,#13301,#13302,#13303),
 .UNSPECIFIED.,.F.,.F.,(4,4),(11.0717103908866,11.6488871259622),
 .UNSPECIFIED.);
#339=B_SPLINE_CURVE_WITH_KNOTS('',3,(#13307,#13308,#13309,#13310),
 .UNSPECIFIED.,.F.,.F.,(4,4),(0.244984789862841,0.822161524938444),
 .UNSPECIFIED.);
#340=B_SPLINE_CURVE_WITH_KNOTS('',3,(#13328,#13329,#13330,#13331),
 .UNSPECIFIED.,.F.,.F.,(4,4),(-0.838823271103535,-0.244984789862841),
 .UNSPECIFIED.);
#341=B_SPLINE_CURVE_WITH_KNOTS('',3,(#13332,#13333,#13334,#13335),
 .UNSPECIFIED.,.F.,.F.,(4,4),(-0.619909717328002,-0.0121844053928019),
 .UNSPECIFIED.);
#342=B_SPLINE_CURVE_WITH_KNOTS('',3,(#13415,#13416,#13417,#13418),
 .UNSPECIFIED.,.F.,.F.,(4,4),(0.011877999214525,0.618764321025346),
 .UNSPECIFIED.);
#343=B_SPLINE_CURVE_WITH_KNOTS('',3,(#13439,#13440,#13441,#13442),
 .UNSPECIFIED.,.F.,.F.,(4,4),(-0.618764321025346,-0.0118779992145249),
 .UNSPECIFIED.);
#344=B_SPLINE_CURVE_WITH_KNOTS('',3,(#13528,#13529,#13530,#13531),
 .UNSPECIFIED.,.F.,.F.,(4,4),(-1.34441069388203E-17,0.619909717328002),
 .UNSPECIFIED.);
#345=B_SPLINE_CURVE_WITH_KNOTS('',3,(#13532,#13533,#13534,#13535),
 .UNSPECIFIED.,.F.,.F.,(4,4),(-0.619909717328002,-0.00253319281730041),
 .UNSPECIFIED.);
#346=B_SPLINE_CURVE_WITH_KNOTS('',3,(#13576,#13577,#13578,#13579,#13580,
#13581),.UNSPECIFIED.,.F.,.F.,(4,1,1,4),(-11.6488871259622,-8.39802760073243,
-5.14716807550265,-0.270878787657975),.UNSPECIFIED.);
#347=B_SPLINE_CURVE_WITH_KNOTS('',3,(#13582,#13583,#13584,#13585,#13586,
#13587),.UNSPECIFIED.,.F.,.F.,(4,1,1,4),(0.270878787657975,5.14716807550265,
8.39802760073243,11.6488871259622),.UNSPECIFIED.);
#348=B_SPLINE_CURVE_WITH_KNOTS('',3,(#13608,#13609,#13610,#13611),
 .UNSPECIFIED.,.F.,.F.,(4,4),(0.0013822243147816,0.618764321025346),
 .UNSPECIFIED.);
#349=B_SPLINE_CURVE_WITH_KNOTS('',3,(#13612,#13613,#13614,#13615),
 .UNSPECIFIED.,.F.,.F.,(4,4),(-0.618764321025346,8.06646416329215E-17),
 .UNSPECIFIED.);
#350=B_SPLINE_CURVE_WITH_KNOTS('',3,(#13636,#13637,#13638,#13639),
 .UNSPECIFIED.,.F.,.F.,(4,4),(-9.36750677027476E-17,0.618764321025346),
 .UNSPECIFIED.);
#351=B_SPLINE_CURVE_WITH_KNOTS('',3,(#13640,#13641,#13642,#13643),
 .UNSPECIFIED.,.F.,.F.,(4,4),(-0.618764321025346,-0.00138222431478148),
 .UNSPECIFIED.);
#352=B_SPLINE_CURVE_WITH_KNOTS('',3,(#13669,#13670,#13671,#13672,#13673),
 .UNSPECIFIED.,.F.,.F.,(4,1,4),(-11.6229931281671,-5.12127407770751,-0.244984789862841),
 .UNSPECIFIED.);
#353=B_SPLINE_CURVE_WITH_KNOTS('',3,(#13674,#13675,#13676,#13677,#13678),
 .UNSPECIFIED.,.F.,.F.,(4,1,4),(0.244984789862841,5.12127407770751,11.6229931281671),
 .UNSPECIFIED.);
#354=B_SPLINE_CURVE_WITH_KNOTS('',3,(#13699,#13700,#13701,#13702),
 .UNSPECIFIED.,.F.,.F.,(4,4),(0.00253319281730024,0.619909717328002),
 .UNSPECIFIED.);
#355=B_SPLINE_CURVE_WITH_KNOTS('',3,(#13703,#13704,#13705,#13706),
 .UNSPECIFIED.,.F.,.F.,(4,4),(-0.619909717328002,-2.51534904016637E-17),
 .UNSPECIFIED.);
#543=SHAPE_REPRESENTATION_RELATIONSHIP('SRR','None',#19523,#553);
#553=ADVANCED_BREP_SHAPE_REPRESENTATION('',(#573),#19466);
#563=STYLED_ITEM('',(#19584),#573);
#573=MANIFOLD_SOLID_BREP('Body1',#7156);
#618=FACE_BOUND('',#1448,.T.);
#619=FACE_BOUND('',#1456,.T.);
#620=FACE_BOUND('',#1467,.T.);
#621=FACE_BOUND('',#1469,.T.);
#622=FACE_BOUND('',#1481,.T.);
#623=FACE_BOUND('',#1490,.T.);
#624=FACE_BOUND('',#1491,.T.);
#625=FACE_BOUND('',#1492,.T.);
#626=FACE_BOUND('',#1507,.T.);
#627=FACE_BOUND('',#1508,.T.);
#628=FACE_BOUND('',#1509,.T.);
#629=FACE_BOUND('',#1545,.T.);
#630=FACE_BOUND('',#1546,.T.);
#631=FACE_BOUND('',#1547,.T.);
#632=FACE_BOUND('',#1548,.T.);
#633=FACE_BOUND('',#1549,.T.);
#634=FACE_BOUND('',#1550,.T.);
#741=PLANE('',#7538);
#742=PLANE('',#7539);
#743=PLANE('',#7540);
#744=PLANE('',#7541);
#745=PLANE('',#7542);
#746=PLANE('',#7543);
#747=PLANE('',#7544);
#748=PLANE('',#7546);
#749=PLANE('',#7547);
#750=PLANE('',#7548);
#751=PLANE('',#7549);
#752=PLANE('',#7550);
#753=PLANE('',#7551);
#754=PLANE('',#7552);
#755=PLANE('',#7558);
#756=PLANE('',#7559);
#757=PLANE('',#7560);
#758=PLANE('',#7561);
#759=PLANE('',#7562);
#760=PLANE('',#7563);
#761=PLANE('',#7564);
#762=PLANE('',#7565);
#763=PLANE('',#7567);
#764=PLANE('',#7569);
#765=PLANE('',#7570);
#766=PLANE('',#7571);
#767=PLANE('',#7572);
#768=PLANE('',#7573);
#769=PLANE('',#7574);
#770=PLANE('',#7575);
#771=PLANE('',#7576);
#772=PLANE('',#7577);
#773=PLANE('',#7578);
#774=PLANE('',#7579);
#775=PLANE('',#7584);
#776=PLANE('',#7586);
#777=PLANE('',#7587);
#778=PLANE('',#7588);
#779=PLANE('',#7589);
#780=PLANE('',#7590);
#781=PLANE('',#7591);
#782=PLANE('',#7592);
#783=PLANE('',#7594);
#784=PLANE('',#7611);
#785=PLANE('',#7630);
#786=PLANE('',#7631);
#787=PLANE('',#7632);
#992=FACE_OUTER_BOUND('',#1437,.T.);
#993=FACE_OUTER_BOUND('',#1438,.T.);
#994=FACE_OUTER_BOUND('',#1439,.T.);
#995=FACE_OUTER_BOUND('',#1440,.T.);
#996=FACE_OUTER_BOUND('',#1441,.T.);
#997=FACE_OUTER_BOUND('',#1442,.T.);
#998=FACE_OUTER_BOUND('',#1443,.T.);
#999=FACE_OUTER_BOUND('',#1444,.T.);
#1000=FACE_OUTER_BOUND('',#1445,.T.);
#1001=FACE_OUTER_BOUND('',#1446,.T.);
#1002=FACE_OUTER_BOUND('',#1447,.T.);
#1003=FACE_OUTER_BOUND('',#1449,.T.);
#1004=FACE_OUTER_BOUND('',#1450,.T.);
#1005=FACE_OUTER_BOUND('',#1451,.T.);
#1006=FACE_OUTER_BOUND('',#1452,.T.);
#1007=FACE_OUTER_BOUND('',#1453,.T.);
#1008=FACE_OUTER_BOUND('',#1454,.T.);
#1009=FACE_OUTER_BOUND('',#1455,.T.);
#1010=FACE_OUTER_BOUND('',#1457,.T.);
#1011=FACE_OUTER_BOUND('',#1458,.T.);
#1012=FACE_OUTER_BOUND('',#1459,.T.);
#1013=FACE_OUTER_BOUND('',#1460,.T.);
#1014=FACE_OUTER_BOUND('',#1461,.T.);
#1015=FACE_OUTER_BOUND('',#1462,.T.);
#1016=FACE_OUTER_BOUND('',#1463,.T.);
#1017=FACE_OUTER_BOUND('',#1464,.T.);
#1018=FACE_OUTER_BOUND('',#1465,.T.);
#1019=FACE_OUTER_BOUND('',#1466,.T.);
#1020=FACE_OUTER_BOUND('',#1468,.T.);
#1021=FACE_OUTER_BOUND('',#1470,.T.);
#1022=FACE_OUTER_BOUND('',#1471,.T.);
#1023=FACE_OUTER_BOUND('',#1472,.T.);
#1024=FACE_OUTER_BOUND('',#1473,.T.);
#1025=FACE_OUTER_BOUND('',#1474,.T.);
#1026=FACE_OUTER_BOUND('',#1475,.T.);
#1027=FACE_OUTER_BOUND('',#1476,.T.);
#1028=FACE_OUTER_BOUND('',#1477,.T.);
#1029=FACE_OUTER_BOUND('',#1478,.T.);
#1030=FACE_OUTER_BOUND('',#1479,.T.);
#1031=FACE_OUTER_BOUND('',#1480,.T.);
#1032=FACE_OUTER_BOUND('',#1482,.T.);
#1033=FACE_OUTER_BOUND('',#1483,.T.);
#1034=FACE_OUTER_BOUND('',#1484,.T.);
#1035=FACE_OUTER_BOUND('',#1485,.T.);
#1036=FACE_OUTER_BOUND('',#1486,.T.);
#1037=FACE_OUTER_BOUND('',#1487,.T.);
#1038=FACE_OUTER_BOUND('',#1488,.T.);
#1039=FACE_OUTER_BOUND('',#1489,.T.);
#1040=FACE_OUTER_BOUND('',#1493,.T.);
#1041=FACE_OUTER_BOUND('',#1494,.T.);
#1042=FACE_OUTER_BOUND('',#1495,.T.);
#1043=FACE_OUTER_BOUND('',#1496,.T.);
#1044=FACE_OUTER_BOUND('',#1497,.T.);
#1045=FACE_OUTER_BOUND('',#1498,.T.);
#1046=FACE_OUTER_BOUND('',#1499,.T.);
#1047=FACE_OUTER_BOUND('',#1500,.T.);
#1048=FACE_OUTER_BOUND('',#1501,.T.);
#1049=FACE_OUTER_BOUND('',#1502,.T.);
#1050=FACE_OUTER_BOUND('',#1503,.T.);
#1051=FACE_OUTER_BOUND('',#1504,.T.);
#1052=FACE_OUTER_BOUND('',#1505,.T.);
#1053=FACE_OUTER_BOUND('',#1506,.T.);
#1054=FACE_OUTER_BOUND('',#1510,.T.);
#1055=FACE_OUTER_BOUND('',#1511,.T.);
#1056=FACE_OUTER_BOUND('',#1512,.T.);
#1057=FACE_OUTER_BOUND('',#1513,.T.);
#1058=FACE_OUTER_BOUND('',#1514,.T.);
#1059=FACE_OUTER_BOUND('',#1515,.T.);
#1060=FACE_OUTER_BOUND('',#1516,.T.);
#1061=FACE_OUTER_BOUND('',#1517,.T.);
#1062=FACE_OUTER_BOUND('',#1518,.T.);
#1063=FACE_OUTER_BOUND('',#1519,.T.);
#1064=FACE_OUTER_BOUND('',#1520,.T.);
#1065=FACE_OUTER_BOUND('',#1521,.T.);
#1066=FACE_OUTER_BOUND('',#1522,.T.);
#1067=FACE_OUTER_BOUND('',#1523,.T.);
#1068=FACE_OUTER_BOUND('',#1524,.T.);
#1069=FACE_OUTER_BOUND('',#1525,.T.);
#1070=FACE_OUTER_BOUND('',#1526,.T.);
#1071=FACE_OUTER_BOUND('',#1527,.T.);
#1072=FACE_OUTER_BOUND('',#1528,.T.);
#1073=FACE_OUTER_BOUND('',#1529,.T.);
#1074=FACE_OUTER_BOUND('',#1530,.T.);
#1075=FACE_OUTER_BOUND('',#1531,.T.);
#1076=FACE_OUTER_BOUND('',#1532,.T.);
#1077=FACE_OUTER_BOUND('',#1533,.T.);
#1078=FACE_OUTER_BOUND('',#1534,.T.);
#1079=FACE_OUTER_BOUND('',#1535,.T.);
#1080=FACE_OUTER_BOUND('',#1536,.T.);
#1081=FACE_OUTER_BOUND('',#1537,.T.);
#1082=FACE_OUTER_BOUND('',#1538,.T.);
#1083=FACE_OUTER_BOUND('',#1539,.T.);
#1084=FACE_OUTER_BOUND('',#1540,.T.);
#1085=FACE_OUTER_BOUND('',#1541,.T.);
#1086=FACE_OUTER_BOUND('',#1542,.T.);
#1087=FACE_OUTER_BOUND('',#1543,.T.);
#1088=FACE_OUTER_BOUND('',#1544,.T.);
#1089=FACE_OUTER_BOUND('',#1551,.T.);
#1090=FACE_OUTER_BOUND('',#1552,.T.);
#1437=EDGE_LOOP('',(#5393,#5394,#5395,#5396));
#1438=EDGE_LOOP('',(#5397,#5398,#5399,#5400));
#1439=EDGE_LOOP('',(#5401,#5402,#5403,#5404));
#1440=EDGE_LOOP('',(#5405,#5406,#5407,#5408));
#1441=EDGE_LOOP('',(#5409,#5410,#5411,#5412));
#1442=EDGE_LOOP('',(#5413,#5414,#5415,#5416));
#1443=EDGE_LOOP('',(#5417,#5418,#5419,#5420));
#1444=EDGE_LOOP('',(#5421,#5422,#5423,#5424));
#1445=EDGE_LOOP('',(#5425,#5426,#5427,#5428));
#1446=EDGE_LOOP('',(#5429,#5430,#5431,#5432));
#1447=EDGE_LOOP('',(#5433,#5434,#5435,#5436,#5437,#5438));
#1448=EDGE_LOOP('',(#5439));
#1449=EDGE_LOOP('',(#5440,#5441,#5442,#5443));
#1450=EDGE_LOOP('',(#5444,#5445,#5446,#5447));
#1451=EDGE_LOOP('',(#5448,#5449,#5450,#5451));
#1452=EDGE_LOOP('',(#5452,#5453,#5454,#5455));
#1453=EDGE_LOOP('',(#5456,#5457,#5458,#5459));
#1454=EDGE_LOOP('',(#5460,#5461,#5462,#5463));
#1455=EDGE_LOOP('',(#5464,#5465,#5466,#5467,#5468,#5469));
#1456=EDGE_LOOP('',(#5470));
#1457=EDGE_LOOP('',(#5471,#5472,#5473,#5474));
#1458=EDGE_LOOP('',(#5475,#5476,#5477,#5478));
#1459=EDGE_LOOP('',(#5479,#5480,#5481,#5482));
#1460=EDGE_LOOP('',(#5483,#5484,#5485,#5486));
#1461=EDGE_LOOP('',(#5487,#5488,#5489,#5490));
#1462=EDGE_LOOP('',(#5491,#5492,#5493,#5494));
#1463=EDGE_LOOP('',(#5495,#5496,#5497,#5498));
#1464=EDGE_LOOP('',(#5499,#5500,#5501,#5502));
#1465=EDGE_LOOP('',(#5503,#5504,#5505,#5506));
#1466=EDGE_LOOP('',(#5507));
#1467=EDGE_LOOP('',(#5508));
#1468=EDGE_LOOP('',(#5509));
#1469=EDGE_LOOP('',(#5510));
#1470=EDGE_LOOP('',(#5511,#5512,#5513,#5514));
#1471=EDGE_LOOP('',(#5515,#5516,#5517,#5518));
#1472=EDGE_LOOP('',(#5519,#5520,#5521,#5522));
#1473=EDGE_LOOP('',(#5523,#5524,#5525,#5526));
#1474=EDGE_LOOP('',(#5527,#5528,#5529,#5530));
#1475=EDGE_LOOP('',(#5531,#5532,#5533,#5534,#5535,#5536));
#1476=EDGE_LOOP('',(#5537,#5538,#5539,#5540,#5541,#5542,#5543,#5544,#5545,
#5546));
#1477=EDGE_LOOP('',(#5547,#5548,#5549,#5550,#5551,#5552,#5553,#5554,#5555,
#5556));
#1478=EDGE_LOOP('',(#5557,#5558,#5559,#5560,#5561,#5562,#5563,#5564,#5565,
#5566));
#1479=EDGE_LOOP('',(#5567,#5568,#5569,#5570,#5571,#5572,#5573,#5574));
#1480=EDGE_LOOP('',(#5575,#5576,#5577,#5578,#5579,#5580,#5581,#5582,#5583,
#5584,#5585,#5586,#5587,#5588,#5589,#5590,#5591,#5592,#5593,#5594,#5595,
#5596,#5597,#5598,#5599,#5600,#5601,#5602,#5603,#5604,#5605,#5606,#5607,
#5608,#5609,#5610,#5611,#5612,#5613,#5614,#5615,#5616));
#1481=EDGE_LOOP('',(#5617,#5618,#5619,#5620,#5621,#5622));
#1482=EDGE_LOOP('',(#5623,#5624,#5625,#5626));
#1483=EDGE_LOOP('',(#5627,#5628,#5629,#5630));
#1484=EDGE_LOOP('',(#5631,#5632,#5633,#5634,#5635,#5636));
#1485=EDGE_LOOP('',(#5637,#5638,#5639,#5640));
#1486=EDGE_LOOP('',(#5641,#5642,#5643,#5644));
#1487=EDGE_LOOP('',(#5645,#5646,#5647,#5648));
#1488=EDGE_LOOP('',(#5649,#5650,#5651,#5652));
#1489=EDGE_LOOP('',(#5653,#5654,#5655,#5656));
#1490=EDGE_LOOP('',(#5657));
#1491=EDGE_LOOP('',(#5658));
#1492=EDGE_LOOP('',(#5659));
#1493=EDGE_LOOP('',(#5660,#5661,#5662,#5663));
#1494=EDGE_LOOP('',(#5664,#5665,#5666,#5667));
#1495=EDGE_LOOP('',(#5668,#5669,#5670,#5671));
#1496=EDGE_LOOP('',(#5672,#5673,#5674,#5675));
#1497=EDGE_LOOP('',(#5676,#5677,#5678,#5679,#5680,#5681,#5682,#5683,#5684,
#5685));
#1498=EDGE_LOOP('',(#5686,#5687,#5688,#5689));
#1499=EDGE_LOOP('',(#5690,#5691,#5692,#5693));
#1500=EDGE_LOOP('',(#5694,#5695,#5696,#5697));
#1501=EDGE_LOOP('',(#5698,#5699,#5700,#5701));
#1502=EDGE_LOOP('',(#5702,#5703,#5704,#5705));
#1503=EDGE_LOOP('',(#5706,#5707,#5708,#5709,#5710,#5711,#5712,#5713,#5714,
#5715));
#1504=EDGE_LOOP('',(#5716,#5717,#5718,#5719));
#1505=EDGE_LOOP('',(#5720,#5721,#5722,#5723));
#1506=EDGE_LOOP('',(#5724,#5725,#5726,#5727));
#1507=EDGE_LOOP('',(#5728));
#1508=EDGE_LOOP('',(#5729));
#1509=EDGE_LOOP('',(#5730));
#1510=EDGE_LOOP('',(#5731,#5732,#5733,#5734));
#1511=EDGE_LOOP('',(#5735,#5736,#5737,#5738));
#1512=EDGE_LOOP('',(#5739,#5740,#5741,#5742,#5743,#5744,#5745,#5746,#5747,
#5748));
#1513=EDGE_LOOP('',(#5749,#5750,#5751,#5752));
#1514=EDGE_LOOP('',(#5753,#5754,#5755,#5756));
#1515=EDGE_LOOP('',(#5757,#5758,#5759,#5760));
#1516=EDGE_LOOP('',(#5761,#5762,#5763,#5764));
#1517=EDGE_LOOP('',(#5765,#5766,#5767,#5768));
#1518=EDGE_LOOP('',(#5769,#5770,#5771));
#1519=EDGE_LOOP('',(#5772,#5773,#5774));
#1520=EDGE_LOOP('',(#5775,#5776,#5777));
#1521=EDGE_LOOP('',(#5778,#5779,#5780,#5781));
#1522=EDGE_LOOP('',(#5782,#5783,#5784,#5785));
#1523=EDGE_LOOP('',(#5786,#5787,#5788));
#1524=EDGE_LOOP('',(#5789,#5790,#5791,#5792));
#1525=EDGE_LOOP('',(#5793,#5794,#5795,#5796));
#1526=EDGE_LOOP('',(#5797,#5798,#5799,#5800));
#1527=EDGE_LOOP('',(#5801,#5802,#5803,#5804));
#1528=EDGE_LOOP('',(#5805,#5806,#5807,#5808));
#1529=EDGE_LOOP('',(#5809,#5810,#5811,#5812));
#1530=EDGE_LOOP('',(#5813,#5814,#5815));
#1531=EDGE_LOOP('',(#5816,#5817,#5818));
#1532=EDGE_LOOP('',(#5819,#5820,#5821));
#1533=EDGE_LOOP('',(#5822,#5823,#5824,#5825));
#1534=EDGE_LOOP('',(#5826,#5827,#5828,#5829));
#1535=EDGE_LOOP('',(#5830,#5831,#5832));
#1536=EDGE_LOOP('',(#5833,#5834,#5835,#5836));
#1537=EDGE_LOOP('',(#5837,#5838,#5839,#5840));
#1538=EDGE_LOOP('',(#5841,#5842,#5843,#5844));
#1539=EDGE_LOOP('',(#5845,#5846,#5847,#5848));
#1540=EDGE_LOOP('',(#5849,#5850,#5851,#5852));
#1541=EDGE_LOOP('',(#5853,#5854,#5855,#5856));
#1542=EDGE_LOOP('',(#5857,#5858,#5859,#5860));
#1543=EDGE_LOOP('',(#5861,#5862,#5863,#5864,#5865,#5866,#5867,#5868));
#1544=EDGE_LOOP('',(#5869,#5870,#5871,#5872));
#1545=EDGE_LOOP('',(#5873,#5874,#5875,#5876,#5877,#5878));
#1546=EDGE_LOOP('',(#5879,#5880,#5881,#5882,#5883,#5884));
#1547=EDGE_LOOP('',(#5885));
#1548=EDGE_LOOP('',(#5886));
#1549=EDGE_LOOP('',(#5887));
#1550=EDGE_LOOP('',(#5888));
#1551=EDGE_LOOP('',(#5889,#5890,#5891,#5892));
#1552=EDGE_LOOP('',(#5893,#5894,#5895,#5896));
#1937=LINE('',#11752,#2411);
#1938=LINE('',#11758,#2412);
#1939=LINE('',#11764,#2413);
#1940=LINE('',#11770,#2414);
#1941=LINE('',#11775,#2415);
#1942=LINE('',#11777,#2416);
#1943=LINE('',#11779,#2417);
#1944=LINE('',#11780,#2418);
#1945=LINE('',#11783,#2419);
#1946=LINE('',#11785,#2420);
#1947=LINE('',#11786,#2421);
#1948=LINE('',#11789,#2422);
#1949=LINE('',#11791,#2423);
#1950=LINE('',#11792,#2424);
#1951=LINE('',#11795,#2425);
#1952=LINE('',#11797,#2426);
#1953=LINE('',#11798,#2427);
#1954=LINE('',#11801,#2428);
#1955=LINE('',#11803,#2429);
#1956=LINE('',#11804,#2430);
#1957=LINE('',#11806,#2431);
#1958=LINE('',#11807,#2432);
#1959=LINE('',#11814,#2433);
#1960=LINE('',#11816,#2434);
#1961=LINE('',#11818,#2435);
#1962=LINE('',#11819,#2436);
#1963=LINE('',#11822,#2437);
#1964=LINE('',#11824,#2438);
#1965=LINE('',#11825,#2439);
#1966=LINE('',#11828,#2440);
#1967=LINE('',#11830,#2441);
#1968=LINE('',#11831,#2442);
#1969=LINE('',#11834,#2443);
#1970=LINE('',#11836,#2444);
#1971=LINE('',#11837,#2445);
#1972=LINE('',#11840,#2446);
#1973=LINE('',#11842,#2447);
#1974=LINE('',#11843,#2448);
#1975=LINE('',#11845,#2449);
#1976=LINE('',#11846,#2450);
#1977=LINE('',#11852,#2451);
#1978=LINE('',#11856,#2452);
#1979=LINE('',#11861,#2453);
#1980=LINE('',#11863,#2454);
#1981=LINE('',#11865,#2455);
#1982=LINE('',#11866,#2456);
#1983=LINE('',#11870,#2457);
#1984=LINE('',#11872,#2458);
#1985=LINE('',#11874,#2459);
#1986=LINE('',#11875,#2460);
#1987=LINE('',#11879,#2461);
#1988=LINE('',#11881,#2462);
#1989=LINE('',#11883,#2463);
#1990=LINE('',#11884,#2464);
#1991=LINE('',#11888,#2465);
#1992=LINE('',#11890,#2466);
#1993=LINE('',#11892,#2467);
#1994=LINE('',#11893,#2468);
#1995=LINE('',#11897,#2469);
#1996=LINE('',#11899,#2470);
#1997=LINE('',#11901,#2471);
#1998=LINE('',#11902,#2472);
#1999=LINE('',#11906,#2473);
#2000=LINE('',#11908,#2474);
#2001=LINE('',#11910,#2475);
#2002=LINE('',#11911,#2476);
#2003=LINE('',#11915,#2477);
#2004=LINE('',#11917,#2478);
#2005=LINE('',#11919,#2479);
#2006=LINE('',#11920,#2480);
#2007=LINE('',#11928,#2481);
#2008=LINE('',#11929,#2482);
#2009=LINE('',#11931,#2483);
#2010=LINE('',#11932,#2484);
#2011=LINE('',#11934,#2485);
#2012=LINE('',#11935,#2486);
#2013=LINE('',#11938,#2487);
#2014=LINE('',#11940,#2488);
#2015=LINE('',#11941,#2489);
#2016=LINE('',#11944,#2490);
#2017=LINE('',#11946,#2491);
#2018=LINE('',#11947,#2492);
#2019=LINE('',#11951,#2493);
#2020=LINE('',#11989,#2494);
#2021=LINE('',#12027,#2495);
#2022=LINE('',#12065,#2496);
#2023=LINE('',#12102,#2497);
#2024=LINE('',#12105,#2498);
#2025=LINE('',#12143,#2499);
#2026=LINE('',#12180,#2500);
#2027=LINE('',#12183,#2501);
#2028=LINE('',#12221,#2502);
#2029=LINE('',#12258,#2503);
#2030=LINE('',#12261,#2504);
#2031=LINE('',#12268,#2505);
#2032=LINE('',#12274,#2506);
#2033=LINE('',#12291,#2507);
#2034=LINE('',#12300,#2508);
#2035=LINE('',#12306,#2509);
#2036=LINE('',#12341,#2510);
#2037=LINE('',#12412,#2511);
#2038=LINE('',#12482,#2512);
#2039=LINE('',#12517,#2513);
#2040=LINE('',#12523,#2514);
#2041=LINE('',#12532,#2515);
#2042=LINE('',#12566,#2516);
#2043=LINE('',#12598,#2517);
#2044=LINE('',#12602,#2518);
#2045=LINE('',#12606,#2519);
#2046=LINE('',#12652,#2520);
#2047=LINE('',#12787,#2521);
#2048=LINE('',#12891,#2522);
#2049=LINE('',#13054,#2523);
#2050=LINE('',#13217,#2524);
#2051=LINE('',#13306,#2525);
#2052=LINE('',#13394,#2526);
#2053=LINE('',#13506,#2527);
#2054=LINE('',#13507,#2528);
#2055=LINE('',#13544,#2529);
#2056=LINE('',#13545,#2530);
#2411=VECTOR('',#8559,0.15);
#2412=VECTOR('',#8566,0.15);
#2413=VECTOR('',#8573,0.15);
#2414=VECTOR('',#8580,0.15);
#2415=VECTOR('',#8585,1.);
#2416=VECTOR('',#8586,1.);
#2417=VECTOR('',#8587,1.);
#2418=VECTOR('',#8588,1.);
#2419=VECTOR('',#8591,1.);
#2420=VECTOR('',#8592,1.);
#2421=VECTOR('',#8593,1.);
#2422=VECTOR('',#8596,1.);
#2423=VECTOR('',#8597,1.);
#2424=VECTOR('',#8598,1.);
#2425=VECTOR('',#8601,1.);
#2426=VECTOR('',#8602,1.);
#2427=VECTOR('',#8603,1.);
#2428=VECTOR('',#8606,1.);
#2429=VECTOR('',#8607,1.);
#2430=VECTOR('',#8608,1.);
#2431=VECTOR('',#8611,1.);
#2432=VECTOR('',#8612,1.);
#2433=VECTOR('',#8619,1.);
#2434=VECTOR('',#8620,1.);
#2435=VECTOR('',#8621,1.);
#2436=VECTOR('',#8622,1.);
#2437=VECTOR('',#8625,1.);
#2438=VECTOR('',#8626,1.);
#2439=VECTOR('',#8627,1.);
#2440=VECTOR('',#8630,1.);
#2441=VECTOR('',#8631,1.);
#2442=VECTOR('',#8632,1.);
#2443=VECTOR('',#8635,1.);
#2444=VECTOR('',#8636,1.);
#2445=VECTOR('',#8637,1.);
#2446=VECTOR('',#8640,1.);
#2447=VECTOR('',#8641,1.);
#2448=VECTOR('',#8642,1.);
#2449=VECTOR('',#8645,1.);
#2450=VECTOR('',#8646,1.);
#2451=VECTOR('',#8653,0.17);
#2452=VECTOR('',#8658,0.17);
#2453=VECTOR('',#8663,1.);
#2454=VECTOR('',#8664,1.);
#2455=VECTOR('',#8665,1.);
#2456=VECTOR('',#8666,1.);
#2457=VECTOR('',#8669,1.);
#2458=VECTOR('',#8670,1.);
#2459=VECTOR('',#8671,1.);
#2460=VECTOR('',#8672,1.);
#2461=VECTOR('',#8675,1.);
#2462=VECTOR('',#8676,1.);
#2463=VECTOR('',#8677,1.);
#2464=VECTOR('',#8678,1.);
#2465=VECTOR('',#8681,1.);
#2466=VECTOR('',#8682,1.);
#2467=VECTOR('',#8683,1.);
#2468=VECTOR('',#8684,1.);
#2469=VECTOR('',#8687,1.);
#2470=VECTOR('',#8688,1.);
#2471=VECTOR('',#8689,1.);
#2472=VECTOR('',#8690,1.);
#2473=VECTOR('',#8693,1.);
#2474=VECTOR('',#8694,1.);
#2475=VECTOR('',#8695,1.);
#2476=VECTOR('',#8696,1.);
#2477=VECTOR('',#8699,1.);
#2478=VECTOR('',#8700,1.);
#2479=VECTOR('',#8701,1.);
#2480=VECTOR('',#8702,1.);
#2481=VECTOR('',#8713,1.);
#2482=VECTOR('',#8714,1.);
#2483=VECTOR('',#8717,1.);
#2484=VECTOR('',#8718,1.);
#2485=VECTOR('',#8721,1.);
#2486=VECTOR('',#8722,1.);
#2487=VECTOR('',#8725,1.);
#2488=VECTOR('',#8726,1.);
#2489=VECTOR('',#8727,1.);
#2490=VECTOR('',#8730,1.);
#2491=VECTOR('',#8731,1.);
#2492=VECTOR('',#8732,1.);
#2493=VECTOR('',#8735,1.);
#2494=VECTOR('',#8736,1.);
#2495=VECTOR('',#8739,1.);
#2496=VECTOR('',#8740,1.);
#2497=VECTOR('',#8741,1.);
#2498=VECTOR('',#8744,1.);
#2499=VECTOR('',#8745,1.);
#2500=VECTOR('',#8746,1.);
#2501=VECTOR('',#8749,1.);
#2502=VECTOR('',#8750,1.);
#2503=VECTOR('',#8751,1.);
#2504=VECTOR('',#8754,1.);
#2505=VECTOR('',#8755,1.);
#2506=VECTOR('',#8756,1.);
#2507=VECTOR('',#8759,1.);
#2508=VECTOR('',#8760,1.);
#2509=VECTOR('',#8761,1.);
#2510=VECTOR('',#8762,1.);
#2511=VECTOR('',#8763,1.);
#2512=VECTOR('',#8764,1.);
#2513=VECTOR('',#8765,1.);
#2514=VECTOR('',#8766,1.);
#2515=VECTOR('',#8767,1.);
#2516=VECTOR('',#8768,1.);
#2517=VECTOR('',#8769,1.);
#2518=VECTOR('',#8774,0.4);
#2519=VECTOR('',#8779,0.4);
#2520=VECTOR('',#8782,1.);
#2521=VECTOR('',#8789,1.);
#2522=VECTOR('',#8792,1.);
#2523=VECTOR('',#8797,1.);
#2524=VECTOR('',#8802,1.);
#2525=VECTOR('',#8807,1.);
#2526=VECTOR('',#8840,1.);
#2527=VECTOR('',#8869,1.);
#2528=VECTOR('',#8870,1.);
#2529=VECTOR('',#8881,1.);
#2530=VECTOR('',#8882,1.);
#2763=CIRCLE('',#7527,0.15);
#2764=CIRCLE('',#7528,0.15);
#2765=CIRCLE('',#7530,0.15);
#2766=CIRCLE('',#7531,0.15);
#2767=CIRCLE('',#7533,0.15);
#2768=CIRCLE('',#7534,0.15);
#2769=CIRCLE('',#7536,0.15);
#2770=CIRCLE('',#7537,0.15);
#2771=CIRCLE('',#7545,0.17);
#2772=CIRCLE('',#7553,0.17);
#2773=CIRCLE('',#7555,0.17);
#2774=CIRCLE('',#7557,0.17);
#2775=CIRCLE('',#7566,0.4);
#2776=CIRCLE('',#7568,0.4);
#2777=CIRCLE('',#7581,0.4);
#2778=CIRCLE('',#7583,0.4);
#2779=CIRCLE('',#7585,0.1);
#2780=CIRCLE('',#7593,0.0999999999999994);
#2781=CIRCLE('',#7595,0.0999999999999999);
#2782=CIRCLE('',#7597,0.1);
#2783=CIRCLE('',#7598,0.1);
#2784=CIRCLE('',#7600,0.100000000000001);
#2785=CIRCLE('',#7601,0.100000000000001);
#2786=CIRCLE('',#7602,0.100000000000002);
#2787=CIRCLE('',#7604,0.0999999999999995);
#2788=CIRCLE('',#7605,0.0999999999999991);
#2789=CIRCLE('',#7608,0.100000000000001);
#2790=CIRCLE('',#7609,0.1);
#2791=CIRCLE('',#7613,0.3);
#2792=CIRCLE('',#7614,0.3);
#2793=CIRCLE('',#7615,0.3);
#2794=CIRCLE('',#7617,0.3);
#2795=CIRCLE('',#7618,0.300000000000002);
#2796=CIRCLE('',#7619,0.3);
#2797=CIRCLE('',#7621,0.3);
#2798=CIRCLE('',#7622,0.299999999999999);
#2799=CIRCLE('',#7623,0.3);
#2800=CIRCLE('',#7626,0.300000000000001);
#2801=CIRCLE('',#7627,0.3);
#2802=CIRCLE('',#7628,0.3);
#3119=VERTEX_POINT('',#11749);
#3120=VERTEX_POINT('',#11751);
#3121=VERTEX_POINT('',#11755);
#3122=VERTEX_POINT('',#11757);
#3123=VERTEX_POINT('',#11761);
#3124=VERTEX_POINT('',#11763);
#3125=VERTEX_POINT('',#11767);
#3126=VERTEX_POINT('',#11769);
#3127=VERTEX_POINT('',#11773);
#3128=VERTEX_POINT('',#11774);
#3129=VERTEX_POINT('',#11776);
#3130=VERTEX_POINT('',#11778);
#3131=VERTEX_POINT('',#11782);
#3132=VERTEX_POINT('',#11784);
#3133=VERTEX_POINT('',#11788);
#3134=VERTEX_POINT('',#11790);
#3135=VERTEX_POINT('',#11794);
#3136=VERTEX_POINT('',#11796);
#3137=VERTEX_POINT('',#11800);
#3138=VERTEX_POINT('',#11802);
#3139=VERTEX_POINT('',#11809);
#3140=VERTEX_POINT('',#11812);
#3141=VERTEX_POINT('',#11813);
#3142=VERTEX_POINT('',#11815);
#3143=VERTEX_POINT('',#11817);
#3144=VERTEX_POINT('',#11821);
#3145=VERTEX_POINT('',#11823);
#3146=VERTEX_POINT('',#11827);
#3147=VERTEX_POINT('',#11829);
#3148=VERTEX_POINT('',#11833);
#3149=VERTEX_POINT('',#11835);
#3150=VERTEX_POINT('',#11839);
#3151=VERTEX_POINT('',#11841);
#3152=VERTEX_POINT('',#11848);
#3153=VERTEX_POINT('',#11851);
#3154=VERTEX_POINT('',#11855);
#3155=VERTEX_POINT('',#11859);
#3156=VERTEX_POINT('',#11860);
#3157=VERTEX_POINT('',#11862);
#3158=VERTEX_POINT('',#11864);
#3159=VERTEX_POINT('',#11868);
#3160=VERTEX_POINT('',#11869);
#3161=VERTEX_POINT('',#11871);
#3162=VERTEX_POINT('',#11873);
#3163=VERTEX_POINT('',#11877);
#3164=VERTEX_POINT('',#11878);
#3165=VERTEX_POINT('',#11880);
#3166=VERTEX_POINT('',#11882);
#3167=VERTEX_POINT('',#11886);
#3168=VERTEX_POINT('',#11887);
#3169=VERTEX_POINT('',#11889);
#3170=VERTEX_POINT('',#11891);
#3171=VERTEX_POINT('',#11895);
#3172=VERTEX_POINT('',#11896);
#3173=VERTEX_POINT('',#11898);
#3174=VERTEX_POINT('',#11900);
#3175=VERTEX_POINT('',#11904);
#3176=VERTEX_POINT('',#11905);
#3177=VERTEX_POINT('',#11907);
#3178=VERTEX_POINT('',#11909);
#3179=VERTEX_POINT('',#11913);
#3180=VERTEX_POINT('',#11914);
#3181=VERTEX_POINT('',#11916);
#3182=VERTEX_POINT('',#11918);
#3183=VERTEX_POINT('',#11922);
#3184=VERTEX_POINT('',#11925);
#3185=VERTEX_POINT('',#11937);
#3186=VERTEX_POINT('',#11939);
#3187=VERTEX_POINT('',#11943);
#3188=VERTEX_POINT('',#11945);
#3189=VERTEX_POINT('',#11949);
#3190=VERTEX_POINT('',#11950);
#3191=VERTEX_POINT('',#11952);
#3192=VERTEX_POINT('',#11959);
#3193=VERTEX_POINT('',#11988);
#3194=VERTEX_POINT('',#11990);
#3195=VERTEX_POINT('',#12026);
#3196=VERTEX_POINT('',#12028);
#3197=VERTEX_POINT('',#12035);
#3198=VERTEX_POINT('',#12064);
#3199=VERTEX_POINT('',#12066);
#3200=VERTEX_POINT('',#12095);
#3201=VERTEX_POINT('',#12104);
#3202=VERTEX_POINT('',#12106);
#3203=VERTEX_POINT('',#12113);
#3204=VERTEX_POINT('',#12142);
#3205=VERTEX_POINT('',#12144);
#3206=VERTEX_POINT('',#12173);
#3207=VERTEX_POINT('',#12182);
#3208=VERTEX_POINT('',#12184);
#3209=VERTEX_POINT('',#12191);
#3210=VERTEX_POINT('',#12220);
#3211=VERTEX_POINT('',#12222);
#3212=VERTEX_POINT('',#12251);
#3213=VERTEX_POINT('',#12260);
#3214=VERTEX_POINT('',#12262);
#3215=VERTEX_POINT('',#12267);
#3216=VERTEX_POINT('',#12269);
#3217=VERTEX_POINT('',#12290);
#3218=VERTEX_POINT('',#12299);
#3219=VERTEX_POINT('',#12305);
#3220=VERTEX_POINT('',#12307);
#3221=VERTEX_POINT('',#12340);
#3222=VERTEX_POINT('',#12342);
#3223=VERTEX_POINT('',#12374);
#3224=VERTEX_POINT('',#12379);
#3225=VERTEX_POINT('',#12411);
#3226=VERTEX_POINT('',#12413);
#3227=VERTEX_POINT('',#12445);
#3228=VERTEX_POINT('',#12450);
#3229=VERTEX_POINT('',#12483);
#3230=VERTEX_POINT('',#12512);
#3231=VERTEX_POINT('',#12518);
#3232=VERTEX_POINT('',#12524);
#3233=VERTEX_POINT('',#12533);
#3234=VERTEX_POINT('',#12534);
#3235=VERTEX_POINT('',#12539);
#3236=VERTEX_POINT('',#12565);
#3237=VERTEX_POINT('',#12567);
#3238=VERTEX_POINT('',#12593);
#3239=VERTEX_POINT('',#12600);
#3240=VERTEX_POINT('',#12604);
#3241=VERTEX_POINT('',#12608);
#3242=VERTEX_POINT('',#12615);
#3243=VERTEX_POINT('',#12622);
#3244=VERTEX_POINT('',#12651);
#3245=VERTEX_POINT('',#12717);
#3246=VERTEX_POINT('',#12770);
#3247=VERTEX_POINT('',#12782);
#3248=VERTEX_POINT('',#12844);
#3249=VERTEX_POINT('',#12854);
#3250=VERTEX_POINT('',#12861);
#3251=VERTEX_POINT('',#12890);
#3252=VERTEX_POINT('',#12892);
#3253=VERTEX_POINT('',#13017);
#3254=VERTEX_POINT('',#13024);
#3255=VERTEX_POINT('',#13053);
#3256=VERTEX_POINT('',#13055);
#3257=VERTEX_POINT('',#13180);
#3258=VERTEX_POINT('',#13187);
#3259=VERTEX_POINT('',#13216);
#3260=VERTEX_POINT('',#13218);
#3261=VERTEX_POINT('',#13269);
#3262=VERTEX_POINT('',#13298);
#3263=VERTEX_POINT('',#13305);
#3264=VERTEX_POINT('',#13327);
#3265=VERTEX_POINT('',#13362);
#3266=VERTEX_POINT('',#13390);
#3267=VERTEX_POINT('',#13485);
#3268=VERTEX_POINT('',#13486);
#3269=VERTEX_POINT('',#13488);
#3270=VERTEX_POINT('',#13492);
#3271=VERTEX_POINT('',#13493);
#3272=VERTEX_POINT('',#13495);
#3273=VERTEX_POINT('',#13499);
#3274=VERTEX_POINT('',#13500);
#3275=VERTEX_POINT('',#13502);
#3276=VERTEX_POINT('',#13537);
#3277=VERTEX_POINT('',#13538);
#3278=VERTEX_POINT('',#13540);
#3937=EDGE_CURVE('',#3119,#3119,#2763,.T.);
#3938=EDGE_CURVE('',#3119,#3120,#1937,.T.);
#3939=EDGE_CURVE('',#3120,#3120,#2764,.T.);
#3940=EDGE_CURVE('',#3121,#3121,#2765,.T.);
#3941=EDGE_CURVE('',#3121,#3122,#1938,.T.);
#3942=EDGE_CURVE('',#3122,#3122,#2766,.T.);
#3943=EDGE_CURVE('',#3123,#3123,#2767,.T.);
#3944=EDGE_CURVE('',#3123,#3124,#1939,.T.);
#3945=EDGE_CURVE('',#3124,#3124,#2768,.T.);
#3946=EDGE_CURVE('',#3125,#3125,#2769,.T.);
#3947=EDGE_CURVE('',#3125,#3126,#1940,.T.);
#3948=EDGE_CURVE('',#3126,#3126,#2770,.T.);
#3949=EDGE_CURVE('',#3127,#3128,#1941,.T.);
#3950=EDGE_CURVE('',#3127,#3129,#1942,.T.);
#3951=EDGE_CURVE('',#3129,#3130,#1943,.T.);
#3952=EDGE_CURVE('',#3128,#3130,#1944,.T.);
#3953=EDGE_CURVE('',#3131,#3127,#1945,.T.);
#3954=EDGE_CURVE('',#3131,#3132,#1946,.T.);
#3955=EDGE_CURVE('',#3132,#3129,#1947,.T.);
#3956=EDGE_CURVE('',#3133,#3131,#1948,.T.);
#3957=EDGE_CURVE('',#3133,#3134,#1949,.T.);
#3958=EDGE_CURVE('',#3134,#3132,#1950,.T.);
#3959=EDGE_CURVE('',#3135,#3133,#1951,.T.);
#3960=EDGE_CURVE('',#3135,#3136,#1952,.T.);
#3961=EDGE_CURVE('',#3136,#3134,#1953,.T.);
#3962=EDGE_CURVE('',#3137,#3135,#1954,.T.);
#3963=EDGE_CURVE('',#3137,#3138,#1955,.T.);
#3964=EDGE_CURVE('',#3138,#3136,#1956,.T.);
#3965=EDGE_CURVE('',#3128,#3137,#1957,.T.);
#3966=EDGE_CURVE('',#3130,#3138,#1958,.T.);
#3967=EDGE_CURVE('',#3139,#3139,#2771,.T.);
#3968=EDGE_CURVE('',#3140,#3141,#1959,.T.);
#3969=EDGE_CURVE('',#3140,#3142,#1960,.T.);
#3970=EDGE_CURVE('',#3142,#3143,#1961,.T.);
#3971=EDGE_CURVE('',#3141,#3143,#1962,.T.);
#3972=EDGE_CURVE('',#3144,#3140,#1963,.T.);
#3973=EDGE_CURVE('',#3144,#3145,#1964,.T.);
#3974=EDGE_CURVE('',#3145,#3142,#1965,.T.);
#3975=EDGE_CURVE('',#3146,#3144,#1966,.T.);
#3976=EDGE_CURVE('',#3146,#3147,#1967,.T.);
#3977=EDGE_CURVE('',#3147,#3145,#1968,.T.);
#3978=EDGE_CURVE('',#3148,#3146,#1969,.T.);
#3979=EDGE_CURVE('',#3148,#3149,#1970,.T.);
#3980=EDGE_CURVE('',#3149,#3147,#1971,.T.);
#3981=EDGE_CURVE('',#3150,#3148,#1972,.T.);
#3982=EDGE_CURVE('',#3150,#3151,#1973,.T.);
#3983=EDGE_CURVE('',#3151,#3149,#1974,.T.);
#3984=EDGE_CURVE('',#3141,#3150,#1975,.T.);
#3985=EDGE_CURVE('',#3143,#3151,#1976,.T.);
#3986=EDGE_CURVE('',#3152,#3152,#2772,.T.);
#3987=EDGE_CURVE('',#3152,#3153,#1977,.T.);
#3988=EDGE_CURVE('',#3153,#3153,#2773,.T.);
#3989=EDGE_CURVE('',#3139,#3154,#1978,.T.);
#3990=EDGE_CURVE('',#3154,#3154,#2774,.T.);
#3991=EDGE_CURVE('',#3155,#3156,#1979,.T.);
#3992=EDGE_CURVE('',#3157,#3155,#1980,.T.);
#3993=EDGE_CURVE('',#3158,#3157,#1981,.T.);
#3994=EDGE_CURVE('',#3158,#3156,#1982,.T.);
#3995=EDGE_CURVE('',#3159,#3160,#1983,.T.);
#3996=EDGE_CURVE('',#3159,#3161,#1984,.T.);
#3997=EDGE_CURVE('',#3162,#3161,#1985,.T.);
#3998=EDGE_CURVE('',#3160,#3162,#1986,.T.);
#3999=EDGE_CURVE('',#3163,#3164,#1987,.T.);
#4000=EDGE_CURVE('',#3163,#3165,#1988,.T.);
#4001=EDGE_CURVE('',#3166,#3165,#1989,.T.);
#4002=EDGE_CURVE('',#3164,#3166,#1990,.T.);
#4003=EDGE_CURVE('',#3167,#3168,#1991,.T.);
#4004=EDGE_CURVE('',#3167,#3169,#1992,.T.);
#4005=EDGE_CURVE('',#3170,#3169,#1993,.T.);
#4006=EDGE_CURVE('',#3168,#3170,#1994,.T.);
#4007=EDGE_CURVE('',#3171,#3172,#1995,.T.);
#4008=EDGE_CURVE('',#3171,#3173,#1996,.T.);
#4009=EDGE_CURVE('',#3174,#3173,#1997,.T.);
#4010=EDGE_CURVE('',#3172,#3174,#1998,.T.);
#4011=EDGE_CURVE('',#3175,#3176,#1999,.T.);
#4012=EDGE_CURVE('',#3177,#3175,#2000,.T.);
#4013=EDGE_CURVE('',#3178,#3177,#2001,.T.);
#4014=EDGE_CURVE('',#3178,#3176,#2002,.T.);
#4015=EDGE_CURVE('',#3179,#3180,#2003,.T.);
#4016=EDGE_CURVE('',#3181,#3179,#2004,.T.);
#4017=EDGE_CURVE('',#3182,#3181,#2005,.T.);
#4018=EDGE_CURVE('',#3182,#3180,#2006,.T.);
#4019=EDGE_CURVE('',#3183,#3183,#2775,.T.);
#4020=EDGE_CURVE('',#3184,#3184,#2776,.T.);
#4021=EDGE_CURVE('',#3156,#3171,#2007,.T.);
#4022=EDGE_CURVE('',#3173,#3158,#2008,.T.);
#4023=EDGE_CURVE('',#3176,#3159,#2009,.T.);
#4024=EDGE_CURVE('',#3161,#3178,#2010,.T.);
#4025=EDGE_CURVE('',#3180,#3163,#2011,.T.);
#4026=EDGE_CURVE('',#3165,#3182,#2012,.T.);
#4027=EDGE_CURVE('',#3185,#3167,#2013,.T.);
#4028=EDGE_CURVE('',#3186,#3185,#2014,.T.);
#4029=EDGE_CURVE('',#3169,#3186,#2015,.T.);
#4030=EDGE_CURVE('',#3187,#3185,#2016,.T.);
#4031=EDGE_CURVE('',#3188,#3187,#2017,.T.);
#4032=EDGE_CURVE('',#3186,#3188,#2018,.T.);
#4033=EDGE_CURVE('',#3189,#3190,#2019,.T.);
#4034=EDGE_CURVE('',#3191,#3190,#264,.T.);
#4035=EDGE_CURVE('',#3192,#3191,#265,.T.);
#4036=EDGE_CURVE('',#3193,#3192,#2020,.T.);
#4037=EDGE_CURVE('',#3194,#3193,#266,.T.);
#4038=EDGE_CURVE('',#3189,#3194,#267,.T.);
#4039=EDGE_CURVE('',#3188,#3195,#2021,.T.);
#4040=EDGE_CURVE('',#3196,#3195,#268,.T.);
#4041=EDGE_CURVE('',#3197,#3196,#269,.T.);
#4042=EDGE_CURVE('',#3198,#3197,#2022,.T.);
#4043=EDGE_CURVE('',#3199,#3198,#270,.T.);
#4044=EDGE_CURVE('',#3200,#3199,#271,.T.);
#4045=EDGE_CURVE('',#3200,#3170,#2023,.T.);
#4046=EDGE_CURVE('',#3181,#3201,#2024,.T.);
#4047=EDGE_CURVE('',#3202,#3201,#272,.T.);
#4048=EDGE_CURVE('',#3203,#3202,#273,.T.);
#4049=EDGE_CURVE('',#3204,#3203,#2025,.T.);
#4050=EDGE_CURVE('',#3205,#3204,#274,.T.);
#4051=EDGE_CURVE('',#3206,#3205,#275,.T.);
#4052=EDGE_CURVE('',#3206,#3166,#2026,.T.);
#4053=EDGE_CURVE('',#3177,#3207,#2027,.T.);
#4054=EDGE_CURVE('',#3208,#3207,#276,.T.);
#4055=EDGE_CURVE('',#3209,#3208,#277,.T.);
#4056=EDGE_CURVE('',#3210,#3209,#2028,.T.);
#4057=EDGE_CURVE('',#3211,#3210,#278,.T.);
#4058=EDGE_CURVE('',#3212,#3211,#279,.T.);
#4059=EDGE_CURVE('',#3212,#3162,#2029,.T.);
#4060=EDGE_CURVE('',#3213,#3172,#2030,.T.);
#4061=EDGE_CURVE('',#3213,#3214,#280,.T.);
#4062=EDGE_CURVE('',#3214,#3215,#2031,.T.);
#4063=EDGE_CURVE('',#3215,#3216,#281,.T.);
#4064=EDGE_CURVE('',#3155,#3216,#2032,.T.);
#4065=EDGE_CURVE('',#3200,#3190,#282,.T.);
#4066=EDGE_CURVE('',#3189,#3195,#283,.T.);
#4067=EDGE_CURVE('',#3217,#3187,#2033,.T.);
#4068=EDGE_CURVE('',#3217,#3201,#284,.T.);
#4069=EDGE_CURVE('',#3218,#3179,#2034,.T.);
#4070=EDGE_CURVE('',#3218,#3207,#285,.T.);
#4071=EDGE_CURVE('',#3219,#3175,#2035,.T.);
#4072=EDGE_CURVE('',#3219,#3220,#286,.T.);
#4073=EDGE_CURVE('',#3220,#3213,#287,.T.);
#4074=EDGE_CURVE('',#3174,#3221,#2036,.T.);
#4075=EDGE_CURVE('',#3222,#3221,#288,.T.);
#4076=EDGE_CURVE('',#3222,#3223,#289,.T.);
#4077=EDGE_CURVE('',#3224,#3223,#290,.T.);
#4078=EDGE_CURVE('',#3224,#3225,#2037,.T.);
#4079=EDGE_CURVE('',#3226,#3225,#291,.T.);
#4080=EDGE_CURVE('',#3226,#3227,#292,.T.);
#4081=EDGE_CURVE('',#3228,#3227,#293,.T.);
#4082=EDGE_CURVE('',#3228,#3157,#2038,.T.);
#4083=EDGE_CURVE('',#3216,#3229,#294,.T.);
#4084=EDGE_CURVE('',#3229,#3230,#295,.T.);
#4085=EDGE_CURVE('',#3160,#3230,#2039,.T.);
#4086=EDGE_CURVE('',#3212,#3231,#296,.T.);
#4087=EDGE_CURVE('',#3164,#3231,#2040,.T.);
#4088=EDGE_CURVE('',#3206,#3232,#297,.T.);
#4089=EDGE_CURVE('',#3168,#3232,#2041,.T.);
#4090=EDGE_CURVE('',#3233,#3234,#298,.T.);
#4091=EDGE_CURVE('',#3234,#3235,#299,.T.);
#4092=EDGE_CURVE('',#3235,#3236,#2042,.T.);
#4093=EDGE_CURVE('',#3236,#3237,#300,.T.);
#4094=EDGE_CURVE('',#3237,#3238,#301,.T.);
#4095=EDGE_CURVE('',#3233,#3238,#2043,.T.);
#4096=EDGE_CURVE('',#3239,#3239,#2777,.T.);
#4097=EDGE_CURVE('',#3239,#3184,#2044,.T.);
#4098=EDGE_CURVE('',#3240,#3240,#2778,.T.);
#4099=EDGE_CURVE('',#3240,#3183,#2045,.T.);
#4100=EDGE_CURVE('',#3233,#3241,#302,.T.);
#4101=EDGE_CURVE('',#3242,#3238,#303,.T.);
#4102=EDGE_CURVE('',#3243,#3242,#304,.T.);
#4103=EDGE_CURVE('',#3244,#3243,#2046,.T.);
#4104=EDGE_CURVE('',#3241,#3244,#305,.T.);
#4105=EDGE_CURVE('',#3199,#3191,#306,.T.);
#4106=EDGE_CURVE('',#3241,#3245,#307,.T.);
#4107=EDGE_CURVE('',#3245,#3234,#308,.T.);
#4108=EDGE_CURVE('',#3192,#3198,#309,.T.);
#4109=EDGE_CURVE('',#3246,#3244,#310,.T.);
#4110=EDGE_CURVE('',#3245,#3246,#2779,.F.);
#4111=EDGE_CURVE('',#3197,#3193,#311,.T.);
#4112=EDGE_CURVE('',#3243,#3247,#312,.T.);
#4113=EDGE_CURVE('',#3247,#3246,#2047,.T.);
#4114=EDGE_CURVE('',#3194,#3196,#313,.T.);
#4115=EDGE_CURVE('',#3237,#3248,#314,.T.);
#4116=EDGE_CURVE('',#3248,#3242,#315,.T.);
#4117=EDGE_CURVE('',#3249,#3232,#316,.T.);
#4118=EDGE_CURVE('',#3250,#3249,#317,.T.);
#4119=EDGE_CURVE('',#3251,#3250,#2048,.T.);
#4120=EDGE_CURVE('',#3252,#3251,#318,.T.);
#4121=EDGE_CURVE('',#3217,#3252,#319,.T.);
#4122=EDGE_CURVE('',#3205,#3249,#320,.T.);
#4123=EDGE_CURVE('',#3250,#3204,#321,.T.);
#4124=EDGE_CURVE('',#3203,#3251,#322,.T.);
#4125=EDGE_CURVE('',#3252,#3202,#323,.T.);
#4126=EDGE_CURVE('',#3253,#3231,#324,.T.);
#4127=EDGE_CURVE('',#3254,#3253,#325,.T.);
#4128=EDGE_CURVE('',#3255,#3254,#2049,.T.);
#4129=EDGE_CURVE('',#3256,#3255,#326,.T.);
#4130=EDGE_CURVE('',#3218,#3256,#327,.T.);
#4131=EDGE_CURVE('',#3211,#3253,#328,.T.);
#4132=EDGE_CURVE('',#3254,#3210,#329,.T.);
#4133=EDGE_CURVE('',#3209,#3255,#330,.T.);
#4134=EDGE_CURVE('',#3256,#3208,#331,.T.);
#4135=EDGE_CURVE('',#3257,#3230,#332,.T.);
#4136=EDGE_CURVE('',#3258,#3257,#333,.T.);
#4137=EDGE_CURVE('',#3259,#3258,#2050,.T.);
#4138=EDGE_CURVE('',#3260,#3259,#334,.T.);
#4139=EDGE_CURVE('',#3219,#3260,#335,.T.);
#4140=EDGE_CURVE('',#3229,#3261,#336,.T.);
#4141=EDGE_CURVE('',#3261,#3257,#337,.T.);
#4142=EDGE_CURVE('',#3262,#3261,#2780,.F.);
#4143=EDGE_CURVE('',#3258,#3262,#338,.T.);
#4144=EDGE_CURVE('',#3262,#3263,#2051,.T.);
#4145=EDGE_CURVE('',#3263,#3259,#339,.T.);
#4146=EDGE_CURVE('',#3260,#3264,#340,.T.);
#4147=EDGE_CURVE('',#3264,#3220,#341,.T.);
#4148=EDGE_CURVE('',#3264,#3263,#2781,.F.);
#4149=EDGE_CURVE('',#3263,#3214,#2782,.F.);
#4150=EDGE_CURVE('',#3214,#3264,#2783,.F.);
#4151=EDGE_CURVE('',#3247,#3248,#2784,.F.);
#4152=EDGE_CURVE('',#3248,#3265,#2785,.F.);
#4153=EDGE_CURVE('',#3265,#3247,#2786,.F.);
#4154=EDGE_CURVE('',#3261,#3215,#2787,.F.);
#4155=EDGE_CURVE('',#3215,#3262,#2788,.F.);
#4156=EDGE_CURVE('',#3266,#3245,#2789,.F.);
#4157=EDGE_CURVE('',#3246,#3266,#2790,.F.);
#4158=EDGE_CURVE('',#3266,#3265,#2052,.T.);
#4159=EDGE_CURVE('',#3235,#3266,#342,.T.);
#4160=EDGE_CURVE('',#3265,#3236,#343,.T.);
#4161=EDGE_CURVE('',#3267,#3268,#2791,.F.);
#4162=EDGE_CURVE('',#3269,#3267,#2792,.F.);
#4163=EDGE_CURVE('',#3268,#3269,#2793,.F.);
#4164=EDGE_CURVE('',#3270,#3271,#2794,.F.);
#4165=EDGE_CURVE('',#3272,#3270,#2795,.F.);
#4166=EDGE_CURVE('',#3271,#3272,#2796,.F.);
#4167=EDGE_CURVE('',#3273,#3274,#2797,.F.);
#4168=EDGE_CURVE('',#3275,#3273,#2798,.F.);
#4169=EDGE_CURVE('',#3274,#3275,#2799,.F.);
#4170=EDGE_CURVE('',#3268,#3275,#2053,.T.);
#4171=EDGE_CURVE('',#3273,#3267,#2054,.T.);
#4172=EDGE_CURVE('',#3227,#3274,#344,.T.);
#4173=EDGE_CURVE('',#3275,#3228,#345,.T.);
#4174=EDGE_CURVE('',#3276,#3277,#2800,.F.);
#4175=EDGE_CURVE('',#3278,#3276,#2801,.F.);
#4176=EDGE_CURVE('',#3277,#3278,#2802,.F.);
#4177=EDGE_CURVE('',#3276,#3272,#2055,.T.);
#4178=EDGE_CURVE('',#3270,#3278,#2056,.T.);
#4179=EDGE_CURVE('',#3274,#3277,#346,.T.);
#4180=EDGE_CURVE('',#3278,#3273,#347,.T.);
#4181=EDGE_CURVE('',#3225,#3276,#348,.T.);
#4182=EDGE_CURVE('',#3277,#3226,#349,.T.);
#4183=EDGE_CURVE('',#3223,#3271,#350,.T.);
#4184=EDGE_CURVE('',#3272,#3224,#351,.T.);
#4185=EDGE_CURVE('',#3271,#3269,#352,.T.);
#4186=EDGE_CURVE('',#3267,#3270,#353,.T.);
#4187=EDGE_CURVE('',#3221,#3268,#354,.T.);
#4188=EDGE_CURVE('',#3269,#3222,#355,.T.);
#5393=ORIENTED_EDGE('',*,*,#3937,.F.);
#5394=ORIENTED_EDGE('',*,*,#3938,.T.);
#5395=ORIENTED_EDGE('',*,*,#3939,.F.);
#5396=ORIENTED_EDGE('',*,*,#3938,.F.);
#5397=ORIENTED_EDGE('',*,*,#3940,.F.);
#5398=ORIENTED_EDGE('',*,*,#3941,.T.);
#5399=ORIENTED_EDGE('',*,*,#3942,.F.);
#5400=ORIENTED_EDGE('',*,*,#3941,.F.);
#5401=ORIENTED_EDGE('',*,*,#3943,.F.);
#5402=ORIENTED_EDGE('',*,*,#3944,.T.);
#5403=ORIENTED_EDGE('',*,*,#3945,.F.);
#5404=ORIENTED_EDGE('',*,*,#3944,.F.);
#5405=ORIENTED_EDGE('',*,*,#3946,.F.);
#5406=ORIENTED_EDGE('',*,*,#3947,.T.);
#5407=ORIENTED_EDGE('',*,*,#3948,.F.);
#5408=ORIENTED_EDGE('',*,*,#3947,.F.);
#5409=ORIENTED_EDGE('',*,*,#3949,.F.);
#5410=ORIENTED_EDGE('',*,*,#3950,.T.);
#5411=ORIENTED_EDGE('',*,*,#3951,.T.);
#5412=ORIENTED_EDGE('',*,*,#3952,.F.);
#5413=ORIENTED_EDGE('',*,*,#3953,.F.);
#5414=ORIENTED_EDGE('',*,*,#3954,.T.);
#5415=ORIENTED_EDGE('',*,*,#3955,.T.);
#5416=ORIENTED_EDGE('',*,*,#3950,.F.);
#5417=ORIENTED_EDGE('',*,*,#3956,.F.);
#5418=ORIENTED_EDGE('',*,*,#3957,.T.);
#5419=ORIENTED_EDGE('',*,*,#3958,.T.);
#5420=ORIENTED_EDGE('',*,*,#3954,.F.);
#5421=ORIENTED_EDGE('',*,*,#3959,.F.);
#5422=ORIENTED_EDGE('',*,*,#3960,.T.);
#5423=ORIENTED_EDGE('',*,*,#3961,.T.);
#5424=ORIENTED_EDGE('',*,*,#3957,.F.);
#5425=ORIENTED_EDGE('',*,*,#3962,.F.);
#5426=ORIENTED_EDGE('',*,*,#3963,.T.);
#5427=ORIENTED_EDGE('',*,*,#3964,.T.);
#5428=ORIENTED_EDGE('',*,*,#3960,.F.);
#5429=ORIENTED_EDGE('',*,*,#3965,.F.);
#5430=ORIENTED_EDGE('',*,*,#3952,.T.);
#5431=ORIENTED_EDGE('',*,*,#3966,.T.);
#5432=ORIENTED_EDGE('',*,*,#3963,.F.);
#5433=ORIENTED_EDGE('',*,*,#3966,.F.);
#5434=ORIENTED_EDGE('',*,*,#3951,.F.);
#5435=ORIENTED_EDGE('',*,*,#3955,.F.);
#5436=ORIENTED_EDGE('',*,*,#3958,.F.);
#5437=ORIENTED_EDGE('',*,*,#3961,.F.);
#5438=ORIENTED_EDGE('',*,*,#3964,.F.);
#5439=ORIENTED_EDGE('',*,*,#3967,.F.);
#5440=ORIENTED_EDGE('',*,*,#3968,.F.);
#5441=ORIENTED_EDGE('',*,*,#3969,.T.);
#5442=ORIENTED_EDGE('',*,*,#3970,.T.);
#5443=ORIENTED_EDGE('',*,*,#3971,.F.);
#5444=ORIENTED_EDGE('',*,*,#3972,.F.);
#5445=ORIENTED_EDGE('',*,*,#3973,.T.);
#5446=ORIENTED_EDGE('',*,*,#3974,.T.);
#5447=ORIENTED_EDGE('',*,*,#3969,.F.);
#5448=ORIENTED_EDGE('',*,*,#3975,.F.);
#5449=ORIENTED_EDGE('',*,*,#3976,.T.);
#5450=ORIENTED_EDGE('',*,*,#3977,.T.);
#5451=ORIENTED_EDGE('',*,*,#3973,.F.);
#5452=ORIENTED_EDGE('',*,*,#3978,.F.);
#5453=ORIENTED_EDGE('',*,*,#3979,.T.);
#5454=ORIENTED_EDGE('',*,*,#3980,.T.);
#5455=ORIENTED_EDGE('',*,*,#3976,.F.);
#5456=ORIENTED_EDGE('',*,*,#3981,.F.);
#5457=ORIENTED_EDGE('',*,*,#3982,.T.);
#5458=ORIENTED_EDGE('',*,*,#3983,.T.);
#5459=ORIENTED_EDGE('',*,*,#3979,.F.);
#5460=ORIENTED_EDGE('',*,*,#3984,.F.);
#5461=ORIENTED_EDGE('',*,*,#3971,.T.);
#5462=ORIENTED_EDGE('',*,*,#3985,.T.);
#5463=ORIENTED_EDGE('',*,*,#3982,.F.);
#5464=ORIENTED_EDGE('',*,*,#3985,.F.);
#5465=ORIENTED_EDGE('',*,*,#3970,.F.);
#5466=ORIENTED_EDGE('',*,*,#3974,.F.);
#5467=ORIENTED_EDGE('',*,*,#3977,.F.);
#5468=ORIENTED_EDGE('',*,*,#3980,.F.);
#5469=ORIENTED_EDGE('',*,*,#3983,.F.);
#5470=ORIENTED_EDGE('',*,*,#3986,.F.);
#5471=ORIENTED_EDGE('',*,*,#3986,.T.);
#5472=ORIENTED_EDGE('',*,*,#3987,.T.);
#5473=ORIENTED_EDGE('',*,*,#3988,.F.);
#5474=ORIENTED_EDGE('',*,*,#3987,.F.);
#5475=ORIENTED_EDGE('',*,*,#3967,.T.);
#5476=ORIENTED_EDGE('',*,*,#3989,.T.);
#5477=ORIENTED_EDGE('',*,*,#3990,.F.);
#5478=ORIENTED_EDGE('',*,*,#3989,.F.);
#5479=ORIENTED_EDGE('',*,*,#3991,.F.);
#5480=ORIENTED_EDGE('',*,*,#3992,.F.);
#5481=ORIENTED_EDGE('',*,*,#3993,.F.);
#5482=ORIENTED_EDGE('',*,*,#3994,.T.);
#5483=ORIENTED_EDGE('',*,*,#3995,.F.);
#5484=ORIENTED_EDGE('',*,*,#3996,.T.);
#5485=ORIENTED_EDGE('',*,*,#3997,.F.);
#5486=ORIENTED_EDGE('',*,*,#3998,.F.);
#5487=ORIENTED_EDGE('',*,*,#3999,.F.);
#5488=ORIENTED_EDGE('',*,*,#4000,.T.);
#5489=ORIENTED_EDGE('',*,*,#4001,.F.);
#5490=ORIENTED_EDGE('',*,*,#4002,.F.);
#5491=ORIENTED_EDGE('',*,*,#4003,.F.);
#5492=ORIENTED_EDGE('',*,*,#4004,.T.);
#5493=ORIENTED_EDGE('',*,*,#4005,.F.);
#5494=ORIENTED_EDGE('',*,*,#4006,.F.);
#5495=ORIENTED_EDGE('',*,*,#4007,.F.);
#5496=ORIENTED_EDGE('',*,*,#4008,.T.);
#5497=ORIENTED_EDGE('',*,*,#4009,.F.);
#5498=ORIENTED_EDGE('',*,*,#4010,.F.);
#5499=ORIENTED_EDGE('',*,*,#4011,.F.);
#5500=ORIENTED_EDGE('',*,*,#4012,.F.);
#5501=ORIENTED_EDGE('',*,*,#4013,.F.);
#5502=ORIENTED_EDGE('',*,*,#4014,.T.);
#5503=ORIENTED_EDGE('',*,*,#4015,.F.);
#5504=ORIENTED_EDGE('',*,*,#4016,.F.);
#5505=ORIENTED_EDGE('',*,*,#4017,.F.);
#5506=ORIENTED_EDGE('',*,*,#4018,.T.);
#5507=ORIENTED_EDGE('',*,*,#4019,.F.);
#5508=ORIENTED_EDGE('',*,*,#3988,.T.);
#5509=ORIENTED_EDGE('',*,*,#4020,.F.);
#5510=ORIENTED_EDGE('',*,*,#3990,.T.);
#5511=ORIENTED_EDGE('',*,*,#4021,.F.);
#5512=ORIENTED_EDGE('',*,*,#3994,.F.);
#5513=ORIENTED_EDGE('',*,*,#4022,.F.);
#5514=ORIENTED_EDGE('',*,*,#4008,.F.);
#5515=ORIENTED_EDGE('',*,*,#4023,.F.);
#5516=ORIENTED_EDGE('',*,*,#4014,.F.);
#5517=ORIENTED_EDGE('',*,*,#4024,.F.);
#5518=ORIENTED_EDGE('',*,*,#3996,.F.);
#5519=ORIENTED_EDGE('',*,*,#4025,.F.);
#5520=ORIENTED_EDGE('',*,*,#4018,.F.);
#5521=ORIENTED_EDGE('',*,*,#4026,.F.);
#5522=ORIENTED_EDGE('',*,*,#4000,.F.);
#5523=ORIENTED_EDGE('',*,*,#4027,.F.);
#5524=ORIENTED_EDGE('',*,*,#4028,.F.);
#5525=ORIENTED_EDGE('',*,*,#4029,.F.);
#5526=ORIENTED_EDGE('',*,*,#4004,.F.);
#5527=ORIENTED_EDGE('',*,*,#4030,.F.);
#5528=ORIENTED_EDGE('',*,*,#4031,.F.);
#5529=ORIENTED_EDGE('',*,*,#4032,.F.);
#5530=ORIENTED_EDGE('',*,*,#4028,.T.);
#5531=ORIENTED_EDGE('',*,*,#4033,.T.);
#5532=ORIENTED_EDGE('',*,*,#4034,.F.);
#5533=ORIENTED_EDGE('',*,*,#4035,.F.);
#5534=ORIENTED_EDGE('',*,*,#4036,.F.);
#5535=ORIENTED_EDGE('',*,*,#4037,.F.);
#5536=ORIENTED_EDGE('',*,*,#4038,.F.);
#5537=ORIENTED_EDGE('',*,*,#4005,.T.);
#5538=ORIENTED_EDGE('',*,*,#4029,.T.);
#5539=ORIENTED_EDGE('',*,*,#4032,.T.);
#5540=ORIENTED_EDGE('',*,*,#4039,.T.);
#5541=ORIENTED_EDGE('',*,*,#4040,.F.);
#5542=ORIENTED_EDGE('',*,*,#4041,.F.);
#5543=ORIENTED_EDGE('',*,*,#4042,.F.);
#5544=ORIENTED_EDGE('',*,*,#4043,.F.);
#5545=ORIENTED_EDGE('',*,*,#4044,.F.);
#5546=ORIENTED_EDGE('',*,*,#4045,.T.);
#5547=ORIENTED_EDGE('',*,*,#4001,.T.);
#5548=ORIENTED_EDGE('',*,*,#4026,.T.);
#5549=ORIENTED_EDGE('',*,*,#4017,.T.);
#5550=ORIENTED_EDGE('',*,*,#4046,.T.);
#5551=ORIENTED_EDGE('',*,*,#4047,.F.);
#5552=ORIENTED_EDGE('',*,*,#4048,.F.);
#5553=ORIENTED_EDGE('',*,*,#4049,.F.);
#5554=ORIENTED_EDGE('',*,*,#4050,.F.);
#5555=ORIENTED_EDGE('',*,*,#4051,.F.);
#5556=ORIENTED_EDGE('',*,*,#4052,.T.);
#5557=ORIENTED_EDGE('',*,*,#3997,.T.);
#5558=ORIENTED_EDGE('',*,*,#4024,.T.);
#5559=ORIENTED_EDGE('',*,*,#4013,.T.);
#5560=ORIENTED_EDGE('',*,*,#4053,.T.);
#5561=ORIENTED_EDGE('',*,*,#4054,.F.);
#5562=ORIENTED_EDGE('',*,*,#4055,.F.);
#5563=ORIENTED_EDGE('',*,*,#4056,.F.);
#5564=ORIENTED_EDGE('',*,*,#4057,.F.);
#5565=ORIENTED_EDGE('',*,*,#4058,.F.);
#5566=ORIENTED_EDGE('',*,*,#4059,.T.);
#5567=ORIENTED_EDGE('',*,*,#3991,.T.);
#5568=ORIENTED_EDGE('',*,*,#4021,.T.);
#5569=ORIENTED_EDGE('',*,*,#4007,.T.);
#5570=ORIENTED_EDGE('',*,*,#4060,.F.);
#5571=ORIENTED_EDGE('',*,*,#4061,.T.);
#5572=ORIENTED_EDGE('',*,*,#4062,.T.);
#5573=ORIENTED_EDGE('',*,*,#4063,.T.);
#5574=ORIENTED_EDGE('',*,*,#4064,.F.);
#5575=ORIENTED_EDGE('',*,*,#4006,.T.);
#5576=ORIENTED_EDGE('',*,*,#4045,.F.);
#5577=ORIENTED_EDGE('',*,*,#4065,.T.);
#5578=ORIENTED_EDGE('',*,*,#4033,.F.);
#5579=ORIENTED_EDGE('',*,*,#4066,.T.);
#5580=ORIENTED_EDGE('',*,*,#4039,.F.);
#5581=ORIENTED_EDGE('',*,*,#4031,.T.);
#5582=ORIENTED_EDGE('',*,*,#4067,.F.);
#5583=ORIENTED_EDGE('',*,*,#4068,.T.);
#5584=ORIENTED_EDGE('',*,*,#4046,.F.);
#5585=ORIENTED_EDGE('',*,*,#4016,.T.);
#5586=ORIENTED_EDGE('',*,*,#4069,.F.);
#5587=ORIENTED_EDGE('',*,*,#4070,.T.);
#5588=ORIENTED_EDGE('',*,*,#4053,.F.);
#5589=ORIENTED_EDGE('',*,*,#4012,.T.);
#5590=ORIENTED_EDGE('',*,*,#4071,.F.);
#5591=ORIENTED_EDGE('',*,*,#4072,.T.);
#5592=ORIENTED_EDGE('',*,*,#4073,.T.);
#5593=ORIENTED_EDGE('',*,*,#4060,.T.);
#5594=ORIENTED_EDGE('',*,*,#4010,.T.);
#5595=ORIENTED_EDGE('',*,*,#4074,.T.);
#5596=ORIENTED_EDGE('',*,*,#4075,.F.);
#5597=ORIENTED_EDGE('',*,*,#4076,.T.);
#5598=ORIENTED_EDGE('',*,*,#4077,.F.);
#5599=ORIENTED_EDGE('',*,*,#4078,.T.);
#5600=ORIENTED_EDGE('',*,*,#4079,.F.);
#5601=ORIENTED_EDGE('',*,*,#4080,.T.);
#5602=ORIENTED_EDGE('',*,*,#4081,.F.);
#5603=ORIENTED_EDGE('',*,*,#4082,.T.);
#5604=ORIENTED_EDGE('',*,*,#3992,.T.);
#5605=ORIENTED_EDGE('',*,*,#4064,.T.);
#5606=ORIENTED_EDGE('',*,*,#4083,.T.);
#5607=ORIENTED_EDGE('',*,*,#4084,.T.);
#5608=ORIENTED_EDGE('',*,*,#4085,.F.);
#5609=ORIENTED_EDGE('',*,*,#3998,.T.);
#5610=ORIENTED_EDGE('',*,*,#4059,.F.);
#5611=ORIENTED_EDGE('',*,*,#4086,.T.);
#5612=ORIENTED_EDGE('',*,*,#4087,.F.);
#5613=ORIENTED_EDGE('',*,*,#4002,.T.);
#5614=ORIENTED_EDGE('',*,*,#4052,.F.);
#5615=ORIENTED_EDGE('',*,*,#4088,.T.);
#5616=ORIENTED_EDGE('',*,*,#4089,.F.);
#5617=ORIENTED_EDGE('',*,*,#4090,.T.);
#5618=ORIENTED_EDGE('',*,*,#4091,.T.);
#5619=ORIENTED_EDGE('',*,*,#4092,.T.);
#5620=ORIENTED_EDGE('',*,*,#4093,.T.);
#5621=ORIENTED_EDGE('',*,*,#4094,.T.);
#5622=ORIENTED_EDGE('',*,*,#4095,.F.);
#5623=ORIENTED_EDGE('',*,*,#4096,.F.);
#5624=ORIENTED_EDGE('',*,*,#4097,.T.);
#5625=ORIENTED_EDGE('',*,*,#4020,.T.);
#5626=ORIENTED_EDGE('',*,*,#4097,.F.);
#5627=ORIENTED_EDGE('',*,*,#4098,.F.);
#5628=ORIENTED_EDGE('',*,*,#4099,.T.);
#5629=ORIENTED_EDGE('',*,*,#4019,.T.);
#5630=ORIENTED_EDGE('',*,*,#4099,.F.);
#5631=ORIENTED_EDGE('',*,*,#4100,.F.);
#5632=ORIENTED_EDGE('',*,*,#4095,.T.);
#5633=ORIENTED_EDGE('',*,*,#4101,.F.);
#5634=ORIENTED_EDGE('',*,*,#4102,.F.);
#5635=ORIENTED_EDGE('',*,*,#4103,.F.);
#5636=ORIENTED_EDGE('',*,*,#4104,.F.);
#5637=ORIENTED_EDGE('',*,*,#4034,.T.);
#5638=ORIENTED_EDGE('',*,*,#4065,.F.);
#5639=ORIENTED_EDGE('',*,*,#4044,.T.);
#5640=ORIENTED_EDGE('',*,*,#4105,.T.);
#5641=ORIENTED_EDGE('',*,*,#4100,.T.);
#5642=ORIENTED_EDGE('',*,*,#4106,.T.);
#5643=ORIENTED_EDGE('',*,*,#4107,.T.);
#5644=ORIENTED_EDGE('',*,*,#4090,.F.);
#5645=ORIENTED_EDGE('',*,*,#4035,.T.);
#5646=ORIENTED_EDGE('',*,*,#4105,.F.);
#5647=ORIENTED_EDGE('',*,*,#4043,.T.);
#5648=ORIENTED_EDGE('',*,*,#4108,.F.);
#5649=ORIENTED_EDGE('',*,*,#4104,.T.);
#5650=ORIENTED_EDGE('',*,*,#4109,.F.);
#5651=ORIENTED_EDGE('',*,*,#4110,.F.);
#5652=ORIENTED_EDGE('',*,*,#4106,.F.);
#5653=ORIENTED_EDGE('',*,*,#4036,.T.);
#5654=ORIENTED_EDGE('',*,*,#4108,.T.);
#5655=ORIENTED_EDGE('',*,*,#4042,.T.);
#5656=ORIENTED_EDGE('',*,*,#4111,.T.);
#5657=ORIENTED_EDGE('',*,*,#3939,.T.);
#5658=ORIENTED_EDGE('',*,*,#3948,.T.);
#5659=ORIENTED_EDGE('',*,*,#4096,.T.);
#5660=ORIENTED_EDGE('',*,*,#4103,.T.);
#5661=ORIENTED_EDGE('',*,*,#4112,.T.);
#5662=ORIENTED_EDGE('',*,*,#4113,.T.);
#5663=ORIENTED_EDGE('',*,*,#4109,.T.);
#5664=ORIENTED_EDGE('',*,*,#4037,.T.);
#5665=ORIENTED_EDGE('',*,*,#4111,.F.);
#5666=ORIENTED_EDGE('',*,*,#4041,.T.);
#5667=ORIENTED_EDGE('',*,*,#4114,.F.);
#5668=ORIENTED_EDGE('',*,*,#4038,.T.);
#5669=ORIENTED_EDGE('',*,*,#4114,.T.);
#5670=ORIENTED_EDGE('',*,*,#4040,.T.);
#5671=ORIENTED_EDGE('',*,*,#4066,.F.);
#5672=ORIENTED_EDGE('',*,*,#4101,.T.);
#5673=ORIENTED_EDGE('',*,*,#4094,.F.);
#5674=ORIENTED_EDGE('',*,*,#4115,.T.);
#5675=ORIENTED_EDGE('',*,*,#4116,.T.);
#5676=ORIENTED_EDGE('',*,*,#4003,.T.);
#5677=ORIENTED_EDGE('',*,*,#4089,.T.);
#5678=ORIENTED_EDGE('',*,*,#4117,.F.);
#5679=ORIENTED_EDGE('',*,*,#4118,.F.);
#5680=ORIENTED_EDGE('',*,*,#4119,.F.);
#5681=ORIENTED_EDGE('',*,*,#4120,.F.);
#5682=ORIENTED_EDGE('',*,*,#4121,.F.);
#5683=ORIENTED_EDGE('',*,*,#4067,.T.);
#5684=ORIENTED_EDGE('',*,*,#4030,.T.);
#5685=ORIENTED_EDGE('',*,*,#4027,.T.);
#5686=ORIENTED_EDGE('',*,*,#4117,.T.);
#5687=ORIENTED_EDGE('',*,*,#4088,.F.);
#5688=ORIENTED_EDGE('',*,*,#4051,.T.);
#5689=ORIENTED_EDGE('',*,*,#4122,.T.);
#5690=ORIENTED_EDGE('',*,*,#4118,.T.);
#5691=ORIENTED_EDGE('',*,*,#4122,.F.);
#5692=ORIENTED_EDGE('',*,*,#4050,.T.);
#5693=ORIENTED_EDGE('',*,*,#4123,.F.);
#5694=ORIENTED_EDGE('',*,*,#4119,.T.);
#5695=ORIENTED_EDGE('',*,*,#4123,.T.);
#5696=ORIENTED_EDGE('',*,*,#4049,.T.);
#5697=ORIENTED_EDGE('',*,*,#4124,.T.);
#5698=ORIENTED_EDGE('',*,*,#4120,.T.);
#5699=ORIENTED_EDGE('',*,*,#4124,.F.);
#5700=ORIENTED_EDGE('',*,*,#4048,.T.);
#5701=ORIENTED_EDGE('',*,*,#4125,.F.);
#5702=ORIENTED_EDGE('',*,*,#4121,.T.);
#5703=ORIENTED_EDGE('',*,*,#4125,.T.);
#5704=ORIENTED_EDGE('',*,*,#4047,.T.);
#5705=ORIENTED_EDGE('',*,*,#4068,.F.);
#5706=ORIENTED_EDGE('',*,*,#3999,.T.);
#5707=ORIENTED_EDGE('',*,*,#4087,.T.);
#5708=ORIENTED_EDGE('',*,*,#4126,.F.);
#5709=ORIENTED_EDGE('',*,*,#4127,.F.);
#5710=ORIENTED_EDGE('',*,*,#4128,.F.);
#5711=ORIENTED_EDGE('',*,*,#4129,.F.);
#5712=ORIENTED_EDGE('',*,*,#4130,.F.);
#5713=ORIENTED_EDGE('',*,*,#4069,.T.);
#5714=ORIENTED_EDGE('',*,*,#4015,.T.);
#5715=ORIENTED_EDGE('',*,*,#4025,.T.);
#5716=ORIENTED_EDGE('',*,*,#4126,.T.);
#5717=ORIENTED_EDGE('',*,*,#4086,.F.);
#5718=ORIENTED_EDGE('',*,*,#4058,.T.);
#5719=ORIENTED_EDGE('',*,*,#4131,.T.);
#5720=ORIENTED_EDGE('',*,*,#4127,.T.);
#5721=ORIENTED_EDGE('',*,*,#4131,.F.);
#5722=ORIENTED_EDGE('',*,*,#4057,.T.);
#5723=ORIENTED_EDGE('',*,*,#4132,.F.);
#5724=ORIENTED_EDGE('',*,*,#4128,.T.);
#5725=ORIENTED_EDGE('',*,*,#4132,.T.);
#5726=ORIENTED_EDGE('',*,*,#4056,.T.);
#5727=ORIENTED_EDGE('',*,*,#4133,.T.);
#5728=ORIENTED_EDGE('',*,*,#3942,.T.);
#5729=ORIENTED_EDGE('',*,*,#3945,.T.);
#5730=ORIENTED_EDGE('',*,*,#4098,.T.);
#5731=ORIENTED_EDGE('',*,*,#4129,.T.);
#5732=ORIENTED_EDGE('',*,*,#4133,.F.);
#5733=ORIENTED_EDGE('',*,*,#4055,.T.);
#5734=ORIENTED_EDGE('',*,*,#4134,.F.);
#5735=ORIENTED_EDGE('',*,*,#4130,.T.);
#5736=ORIENTED_EDGE('',*,*,#4134,.T.);
#5737=ORIENTED_EDGE('',*,*,#4054,.T.);
#5738=ORIENTED_EDGE('',*,*,#4070,.F.);
#5739=ORIENTED_EDGE('',*,*,#3995,.T.);
#5740=ORIENTED_EDGE('',*,*,#4085,.T.);
#5741=ORIENTED_EDGE('',*,*,#4135,.F.);
#5742=ORIENTED_EDGE('',*,*,#4136,.F.);
#5743=ORIENTED_EDGE('',*,*,#4137,.F.);
#5744=ORIENTED_EDGE('',*,*,#4138,.F.);
#5745=ORIENTED_EDGE('',*,*,#4139,.F.);
#5746=ORIENTED_EDGE('',*,*,#4071,.T.);
#5747=ORIENTED_EDGE('',*,*,#4011,.T.);
#5748=ORIENTED_EDGE('',*,*,#4023,.T.);
#5749=ORIENTED_EDGE('',*,*,#4135,.T.);
#5750=ORIENTED_EDGE('',*,*,#4084,.F.);
#5751=ORIENTED_EDGE('',*,*,#4140,.T.);
#5752=ORIENTED_EDGE('',*,*,#4141,.T.);
#5753=ORIENTED_EDGE('',*,*,#4136,.T.);
#5754=ORIENTED_EDGE('',*,*,#4141,.F.);
#5755=ORIENTED_EDGE('',*,*,#4142,.F.);
#5756=ORIENTED_EDGE('',*,*,#4143,.F.);
#5757=ORIENTED_EDGE('',*,*,#4137,.T.);
#5758=ORIENTED_EDGE('',*,*,#4143,.T.);
#5759=ORIENTED_EDGE('',*,*,#4144,.T.);
#5760=ORIENTED_EDGE('',*,*,#4145,.T.);
#5761=ORIENTED_EDGE('',*,*,#4139,.T.);
#5762=ORIENTED_EDGE('',*,*,#4146,.T.);
#5763=ORIENTED_EDGE('',*,*,#4147,.T.);
#5764=ORIENTED_EDGE('',*,*,#4072,.F.);
#5765=ORIENTED_EDGE('',*,*,#4138,.T.);
#5766=ORIENTED_EDGE('',*,*,#4145,.F.);
#5767=ORIENTED_EDGE('',*,*,#4148,.F.);
#5768=ORIENTED_EDGE('',*,*,#4146,.F.);
#5769=ORIENTED_EDGE('',*,*,#4149,.T.);
#5770=ORIENTED_EDGE('',*,*,#4150,.T.);
#5771=ORIENTED_EDGE('',*,*,#4148,.T.);
#5772=ORIENTED_EDGE('',*,*,#4151,.T.);
#5773=ORIENTED_EDGE('',*,*,#4152,.T.);
#5774=ORIENTED_EDGE('',*,*,#4153,.T.);
#5775=ORIENTED_EDGE('',*,*,#4142,.T.);
#5776=ORIENTED_EDGE('',*,*,#4154,.T.);
#5777=ORIENTED_EDGE('',*,*,#4155,.T.);
#5778=ORIENTED_EDGE('',*,*,#4149,.F.);
#5779=ORIENTED_EDGE('',*,*,#4144,.F.);
#5780=ORIENTED_EDGE('',*,*,#4155,.F.);
#5781=ORIENTED_EDGE('',*,*,#4062,.F.);
#5782=ORIENTED_EDGE('',*,*,#4083,.F.);
#5783=ORIENTED_EDGE('',*,*,#4063,.F.);
#5784=ORIENTED_EDGE('',*,*,#4154,.F.);
#5785=ORIENTED_EDGE('',*,*,#4140,.F.);
#5786=ORIENTED_EDGE('',*,*,#4156,.T.);
#5787=ORIENTED_EDGE('',*,*,#4110,.T.);
#5788=ORIENTED_EDGE('',*,*,#4157,.T.);
#5789=ORIENTED_EDGE('',*,*,#4157,.F.);
#5790=ORIENTED_EDGE('',*,*,#4113,.F.);
#5791=ORIENTED_EDGE('',*,*,#4153,.F.);
#5792=ORIENTED_EDGE('',*,*,#4158,.F.);
#5793=ORIENTED_EDGE('',*,*,#4091,.F.);
#5794=ORIENTED_EDGE('',*,*,#4107,.F.);
#5795=ORIENTED_EDGE('',*,*,#4156,.F.);
#5796=ORIENTED_EDGE('',*,*,#4159,.F.);
#5797=ORIENTED_EDGE('',*,*,#4093,.F.);
#5798=ORIENTED_EDGE('',*,*,#4160,.F.);
#5799=ORIENTED_EDGE('',*,*,#4152,.F.);
#5800=ORIENTED_EDGE('',*,*,#4115,.F.);
#5801=ORIENTED_EDGE('',*,*,#4102,.T.);
#5802=ORIENTED_EDGE('',*,*,#4116,.F.);
#5803=ORIENTED_EDGE('',*,*,#4151,.F.);
#5804=ORIENTED_EDGE('',*,*,#4112,.F.);
#5805=ORIENTED_EDGE('',*,*,#4073,.F.);
#5806=ORIENTED_EDGE('',*,*,#4147,.F.);
#5807=ORIENTED_EDGE('',*,*,#4150,.F.);
#5808=ORIENTED_EDGE('',*,*,#4061,.F.);
#5809=ORIENTED_EDGE('',*,*,#4159,.T.);
#5810=ORIENTED_EDGE('',*,*,#4158,.T.);
#5811=ORIENTED_EDGE('',*,*,#4160,.T.);
#5812=ORIENTED_EDGE('',*,*,#4092,.F.);
#5813=ORIENTED_EDGE('',*,*,#4161,.F.);
#5814=ORIENTED_EDGE('',*,*,#4162,.F.);
#5815=ORIENTED_EDGE('',*,*,#4163,.F.);
#5816=ORIENTED_EDGE('',*,*,#4164,.F.);
#5817=ORIENTED_EDGE('',*,*,#4165,.F.);
#5818=ORIENTED_EDGE('',*,*,#4166,.F.);
#5819=ORIENTED_EDGE('',*,*,#4167,.F.);
#5820=ORIENTED_EDGE('',*,*,#4168,.F.);
#5821=ORIENTED_EDGE('',*,*,#4169,.F.);
#5822=ORIENTED_EDGE('',*,*,#4161,.T.);
#5823=ORIENTED_EDGE('',*,*,#4170,.T.);
#5824=ORIENTED_EDGE('',*,*,#4168,.T.);
#5825=ORIENTED_EDGE('',*,*,#4171,.T.);
#5826=ORIENTED_EDGE('',*,*,#4081,.T.);
#5827=ORIENTED_EDGE('',*,*,#4172,.T.);
#5828=ORIENTED_EDGE('',*,*,#4169,.T.);
#5829=ORIENTED_EDGE('',*,*,#4173,.T.);
#5830=ORIENTED_EDGE('',*,*,#4174,.F.);
#5831=ORIENTED_EDGE('',*,*,#4175,.F.);
#5832=ORIENTED_EDGE('',*,*,#4176,.F.);
#5833=ORIENTED_EDGE('',*,*,#4175,.T.);
#5834=ORIENTED_EDGE('',*,*,#4177,.T.);
#5835=ORIENTED_EDGE('',*,*,#4165,.T.);
#5836=ORIENTED_EDGE('',*,*,#4178,.T.);
#5837=ORIENTED_EDGE('',*,*,#4167,.T.);
#5838=ORIENTED_EDGE('',*,*,#4179,.T.);
#5839=ORIENTED_EDGE('',*,*,#4176,.T.);
#5840=ORIENTED_EDGE('',*,*,#4180,.T.);
#5841=ORIENTED_EDGE('',*,*,#4079,.T.);
#5842=ORIENTED_EDGE('',*,*,#4181,.T.);
#5843=ORIENTED_EDGE('',*,*,#4174,.T.);
#5844=ORIENTED_EDGE('',*,*,#4182,.T.);
#5845=ORIENTED_EDGE('',*,*,#4077,.T.);
#5846=ORIENTED_EDGE('',*,*,#4183,.T.);
#5847=ORIENTED_EDGE('',*,*,#4166,.T.);
#5848=ORIENTED_EDGE('',*,*,#4184,.T.);
#5849=ORIENTED_EDGE('',*,*,#4164,.T.);
#5850=ORIENTED_EDGE('',*,*,#4185,.T.);
#5851=ORIENTED_EDGE('',*,*,#4162,.T.);
#5852=ORIENTED_EDGE('',*,*,#4186,.T.);
#5853=ORIENTED_EDGE('',*,*,#4075,.T.);
#5854=ORIENTED_EDGE('',*,*,#4187,.T.);
#5855=ORIENTED_EDGE('',*,*,#4163,.T.);
#5856=ORIENTED_EDGE('',*,*,#4188,.T.);
#5857=ORIENTED_EDGE('',*,*,#4182,.F.);
#5858=ORIENTED_EDGE('',*,*,#4179,.F.);
#5859=ORIENTED_EDGE('',*,*,#4172,.F.);
#5860=ORIENTED_EDGE('',*,*,#4080,.F.);
#5861=ORIENTED_EDGE('',*,*,#3993,.T.);
#5862=ORIENTED_EDGE('',*,*,#4082,.F.);
#5863=ORIENTED_EDGE('',*,*,#4173,.F.);
#5864=ORIENTED_EDGE('',*,*,#4170,.F.);
#5865=ORIENTED_EDGE('',*,*,#4187,.F.);
#5866=ORIENTED_EDGE('',*,*,#4074,.F.);
#5867=ORIENTED_EDGE('',*,*,#4009,.T.);
#5868=ORIENTED_EDGE('',*,*,#4022,.T.);
#5869=ORIENTED_EDGE('',*,*,#4178,.F.);
#5870=ORIENTED_EDGE('',*,*,#4186,.F.);
#5871=ORIENTED_EDGE('',*,*,#4171,.F.);
#5872=ORIENTED_EDGE('',*,*,#4180,.F.);
#5873=ORIENTED_EDGE('',*,*,#3968,.T.);
#5874=ORIENTED_EDGE('',*,*,#3984,.T.);
#5875=ORIENTED_EDGE('',*,*,#3981,.T.);
#5876=ORIENTED_EDGE('',*,*,#3978,.T.);
#5877=ORIENTED_EDGE('',*,*,#3975,.T.);
#5878=ORIENTED_EDGE('',*,*,#3972,.T.);
#5879=ORIENTED_EDGE('',*,*,#3949,.T.);
#5880=ORIENTED_EDGE('',*,*,#3965,.T.);
#5881=ORIENTED_EDGE('',*,*,#3962,.T.);
#5882=ORIENTED_EDGE('',*,*,#3959,.T.);
#5883=ORIENTED_EDGE('',*,*,#3956,.T.);
#5884=ORIENTED_EDGE('',*,*,#3953,.T.);
#5885=ORIENTED_EDGE('',*,*,#3946,.T.);
#5886=ORIENTED_EDGE('',*,*,#3943,.T.);
#5887=ORIENTED_EDGE('',*,*,#3940,.T.);
#5888=ORIENTED_EDGE('',*,*,#3937,.T.);
#5889=ORIENTED_EDGE('',*,*,#4183,.F.);
#5890=ORIENTED_EDGE('',*,*,#4076,.F.);
#5891=ORIENTED_EDGE('',*,*,#4188,.F.);
#5892=ORIENTED_EDGE('',*,*,#4185,.F.);
#5893=ORIENTED_EDGE('',*,*,#4181,.F.);
#5894=ORIENTED_EDGE('',*,*,#4078,.F.);
#5895=ORIENTED_EDGE('',*,*,#4184,.F.);
#5896=ORIENTED_EDGE('',*,*,#4177,.F.);
#6641=CYLINDRICAL_SURFACE('',#7526,0.15);
#6642=CYLINDRICAL_SURFACE('',#7529,0.15);
#6643=CYLINDRICAL_SURFACE('',#7532,0.15);
#6644=CYLINDRICAL_SURFACE('',#7535,0.15);
#6645=CYLINDRICAL_SURFACE('',#7554,0.17);
#6646=CYLINDRICAL_SURFACE('',#7556,0.17);
#6647=CYLINDRICAL_SURFACE('',#7580,0.4);
#6648=CYLINDRICAL_SURFACE('',#7582,0.4);
#6649=CYLINDRICAL_SURFACE('',#7606,0.1);
#6650=CYLINDRICAL_SURFACE('',#7610,0.1);
#6651=CYLINDRICAL_SURFACE('',#7624,0.3);
#6652=CYLINDRICAL_SURFACE('',#7629,0.3);
#6914=ADVANCED_FACE('',(#992),#6641,.F.);
#6915=ADVANCED_FACE('',(#993),#6642,.F.);
#6916=ADVANCED_FACE('',(#994),#6643,.F.);
#6917=ADVANCED_FACE('',(#995),#6644,.F.);
#6918=ADVANCED_FACE('',(#996),#741,.F.);
#6919=ADVANCED_FACE('',(#997),#742,.F.);
#6920=ADVANCED_FACE('',(#998),#743,.F.);
#6921=ADVANCED_FACE('',(#999),#744,.F.);
#6922=ADVANCED_FACE('',(#1000),#745,.F.);
#6923=ADVANCED_FACE('',(#1001),#746,.F.);
#6924=ADVANCED_FACE('',(#1002,#618),#747,.F.);
#6925=ADVANCED_FACE('',(#1003),#748,.F.);
#6926=ADVANCED_FACE('',(#1004),#749,.F.);
#6927=ADVANCED_FACE('',(#1005),#750,.F.);
#6928=ADVANCED_FACE('',(#1006),#751,.F.);
#6929=ADVANCED_FACE('',(#1007),#752,.F.);
#6930=ADVANCED_FACE('',(#1008),#753,.F.);
#6931=ADVANCED_FACE('',(#1009,#619),#754,.F.);
#6932=ADVANCED_FACE('',(#1010),#6645,.F.);
#6933=ADVANCED_FACE('',(#1011),#6646,.F.);
#6934=ADVANCED_FACE('',(#1012),#755,.F.);
#6935=ADVANCED_FACE('',(#1013),#756,.F.);
#6936=ADVANCED_FACE('',(#1014),#757,.F.);
#6937=ADVANCED_FACE('',(#1015),#758,.F.);
#6938=ADVANCED_FACE('',(#1016),#759,.F.);
#6939=ADVANCED_FACE('',(#1017),#760,.F.);
#6940=ADVANCED_FACE('',(#1018),#761,.F.);
#6941=ADVANCED_FACE('',(#1019,#620),#762,.F.);
#6942=ADVANCED_FACE('',(#1020,#621),#763,.F.);
#6943=ADVANCED_FACE('',(#1021),#764,.F.);
#6944=ADVANCED_FACE('',(#1022),#765,.F.);
#6945=ADVANCED_FACE('',(#1023),#766,.F.);
#6946=ADVANCED_FACE('',(#1024),#767,.F.);
#6947=ADVANCED_FACE('',(#1025),#768,.F.);
#6948=ADVANCED_FACE('',(#1026),#769,.T.);
#6949=ADVANCED_FACE('',(#1027),#770,.T.);
#6950=ADVANCED_FACE('',(#1028),#771,.T.);
#6951=ADVANCED_FACE('',(#1029),#772,.T.);
#6952=ADVANCED_FACE('',(#1030),#773,.T.);
#6953=ADVANCED_FACE('',(#1031,#622),#774,.F.);
#6954=ADVANCED_FACE('',(#1032),#6647,.T.);
#6955=ADVANCED_FACE('',(#1033),#6648,.T.);
#6956=ADVANCED_FACE('',(#1034),#775,.T.);
#6957=ADVANCED_FACE('',(#1035),#124,.T.);
#6958=ADVANCED_FACE('',(#1036),#125,.T.);
#6959=ADVANCED_FACE('',(#1037),#126,.T.);
#6960=ADVANCED_FACE('',(#1038),#127,.T.);
#6961=ADVANCED_FACE('',(#1039,#623,#624,#625),#776,.F.);
#6962=ADVANCED_FACE('',(#1040),#777,.F.);
#6963=ADVANCED_FACE('',(#1041),#128,.T.);
#6964=ADVANCED_FACE('',(#1042),#129,.T.);
#6965=ADVANCED_FACE('',(#1043),#130,.T.);
#6966=ADVANCED_FACE('',(#1044),#778,.T.);
#6967=ADVANCED_FACE('',(#1045),#131,.T.);
#6968=ADVANCED_FACE('',(#1046),#132,.T.);
#6969=ADVANCED_FACE('',(#1047),#779,.F.);
#6970=ADVANCED_FACE('',(#1048),#133,.T.);
#6971=ADVANCED_FACE('',(#1049),#134,.T.);
#6972=ADVANCED_FACE('',(#1050),#780,.T.);
#6973=ADVANCED_FACE('',(#1051),#135,.T.);
#6974=ADVANCED_FACE('',(#1052),#136,.T.);
#6975=ADVANCED_FACE('',(#1053,#626,#627,#628),#781,.F.);
#6976=ADVANCED_FACE('',(#1054),#137,.T.);
#6977=ADVANCED_FACE('',(#1055),#138,.T.);
#6978=ADVANCED_FACE('',(#1056),#782,.T.);
#6979=ADVANCED_FACE('',(#1057),#139,.T.);
#6980=ADVANCED_FACE('',(#1058),#140,.T.);
#6981=ADVANCED_FACE('',(#1059),#783,.F.);
#6982=ADVANCED_FACE('',(#1060),#141,.T.);
#6983=ADVANCED_FACE('',(#1061),#142,.T.);
#6984=ADVANCED_FACE('',(#1062),#84,.F.);
#6985=ADVANCED_FACE('',(#1063),#85,.F.);
#6986=ADVANCED_FACE('',(#1064),#86,.F.);
#6987=ADVANCED_FACE('',(#1065),#6649,.F.);
#6988=ADVANCED_FACE('',(#1066),#143,.T.);
#6989=ADVANCED_FACE('',(#1067),#87,.F.);
#6990=ADVANCED_FACE('',(#1068),#6650,.F.);
#6991=ADVANCED_FACE('',(#1069),#144,.T.);
#6992=ADVANCED_FACE('',(#1070),#145,.T.);
#6993=ADVANCED_FACE('',(#1071),#146,.T.);
#6994=ADVANCED_FACE('',(#1072),#147,.T.);
#6995=ADVANCED_FACE('',(#1073),#784,.T.);
#6996=ADVANCED_FACE('',(#1074),#88,.T.);
#6997=ADVANCED_FACE('',(#1075),#89,.T.);
#6998=ADVANCED_FACE('',(#1076),#90,.T.);
#6999=ADVANCED_FACE('',(#1077),#6651,.T.);
#7000=ADVANCED_FACE('',(#1078),#148,.F.);
#7001=ADVANCED_FACE('',(#1079),#91,.T.);
#7002=ADVANCED_FACE('',(#1080),#6652,.T.);
#7003=ADVANCED_FACE('',(#1081),#149,.F.);
#7004=ADVANCED_FACE('',(#1082),#150,.F.);
#7005=ADVANCED_FACE('',(#1083),#151,.F.);
#7006=ADVANCED_FACE('',(#1084),#152,.F.);
#7007=ADVANCED_FACE('',(#1085),#153,.F.);
#7008=ADVANCED_FACE('',(#1086),#154,.F.);
#7009=ADVANCED_FACE('',(#1087),#785,.F.);
#7010=ADVANCED_FACE('',(#1088,#629,#630,#631,#632,#633,#634),#786,.T.);
#7011=ADVANCED_FACE('',(#1089),#155,.F.);
#7012=ADVANCED_FACE('',(#1090),#787,.F.);
#7156=CLOSED_SHELL('',(#6914,#6915,#6916,#6917,#6918,#6919,#6920,#6921,
#6922,#6923,#6924,#6925,#6926,#6927,#6928,#6929,#6930,#6931,#6932,#6933,
#6934,#6935,#6936,#6937,#6938,#6939,#6940,#6941,#6942,#6943,#6944,#6945,
#6946,#6947,#6948,#6949,#6950,#6951,#6952,#6953,#6954,#6955,#6956,#6957,
#6958,#6959,#6960,#6961,#6962,#6963,#6964,#6965,#6966,#6967,#6968,#6969,
#6970,#6971,#6972,#6973,#6974,#6975,#6976,#6977,#6978,#6979,#6980,#6981,
#6982,#6983,#6984,#6985,#6986,#6987,#6988,#6989,#6990,#6991,#6992,#6993,
#6994,#6995,#6996,#6997,#6998,#6999,#7000,#7001,#7002,#7003,#7004,#7005,
#7006,#7007,#7008,#7009,#7010,#7011,#7012));
#7525=AXIS2_PLACEMENT_3D('',#11747,#8553,#8554);
#7526=AXIS2_PLACEMENT_3D('',#11748,#8555,#8556);
#7527=AXIS2_PLACEMENT_3D('',#11750,#8557,#8558);
#7528=AXIS2_PLACEMENT_3D('',#11753,#8560,#8561);
#7529=AXIS2_PLACEMENT_3D('',#11754,#8562,#8563);
#7530=AXIS2_PLACEMENT_3D('',#11756,#8564,#8565);
#7531=AXIS2_PLACEMENT_3D('',#11759,#8567,#8568);
#7532=AXIS2_PLACEMENT_3D('',#11760,#8569,#8570);
#7533=AXIS2_PLACEMENT_3D('',#11762,#8571,#8572);
#7534=AXIS2_PLACEMENT_3D('',#11765,#8574,#8575);
#7535=AXIS2_PLACEMENT_3D('',#11766,#8576,#8577);
#7536=AXIS2_PLACEMENT_3D('',#11768,#8578,#8579);
#7537=AXIS2_PLACEMENT_3D('',#11771,#8581,#8582);
#7538=AXIS2_PLACEMENT_3D('',#11772,#8583,#8584);
#7539=AXIS2_PLACEMENT_3D('',#11781,#8589,#8590);
#7540=AXIS2_PLACEMENT_3D('',#11787,#8594,#8595);
#7541=AXIS2_PLACEMENT_3D('',#11793,#8599,#8600);
#7542=AXIS2_PLACEMENT_3D('',#11799,#8604,#8605);
#7543=AXIS2_PLACEMENT_3D('',#11805,#8609,#8610);
#7544=AXIS2_PLACEMENT_3D('',#11808,#8613,#8614);
#7545=AXIS2_PLACEMENT_3D('',#11810,#8615,#8616);
#7546=AXIS2_PLACEMENT_3D('',#11811,#8617,#8618);
#7547=AXIS2_PLACEMENT_3D('',#11820,#8623,#8624);
#7548=AXIS2_PLACEMENT_3D('',#11826,#8628,#8629);
#7549=AXIS2_PLACEMENT_3D('',#11832,#8633,#8634);
#7550=AXIS2_PLACEMENT_3D('',#11838,#8638,#8639);
#7551=AXIS2_PLACEMENT_3D('',#11844,#8643,#8644);
#7552=AXIS2_PLACEMENT_3D('',#11847,#8647,#8648);
#7553=AXIS2_PLACEMENT_3D('',#11849,#8649,#8650);
#7554=AXIS2_PLACEMENT_3D('',#11850,#8651,#8652);
#7555=AXIS2_PLACEMENT_3D('',#11853,#8654,#8655);
#7556=AXIS2_PLACEMENT_3D('',#11854,#8656,#8657);
#7557=AXIS2_PLACEMENT_3D('',#11857,#8659,#8660);
#7558=AXIS2_PLACEMENT_3D('',#11858,#8661,#8662);
#7559=AXIS2_PLACEMENT_3D('',#11867,#8667,#8668);
#7560=AXIS2_PLACEMENT_3D('',#11876,#8673,#8674);
#7561=AXIS2_PLACEMENT_3D('',#11885,#8679,#8680);
#7562=AXIS2_PLACEMENT_3D('',#11894,#8685,#8686);
#7563=AXIS2_PLACEMENT_3D('',#11903,#8691,#8692);
#7564=AXIS2_PLACEMENT_3D('',#11912,#8697,#8698);
#7565=AXIS2_PLACEMENT_3D('',#11921,#8703,#8704);
#7566=AXIS2_PLACEMENT_3D('',#11923,#8705,#8706);
#7567=AXIS2_PLACEMENT_3D('',#11924,#8707,#8708);
#7568=AXIS2_PLACEMENT_3D('',#11926,#8709,#8710);
#7569=AXIS2_PLACEMENT_3D('',#11927,#8711,#8712);
#7570=AXIS2_PLACEMENT_3D('',#11930,#8715,#8716);
#7571=AXIS2_PLACEMENT_3D('',#11933,#8719,#8720);
#7572=AXIS2_PLACEMENT_3D('',#11936,#8723,#8724);
#7573=AXIS2_PLACEMENT_3D('',#11942,#8728,#8729);
#7574=AXIS2_PLACEMENT_3D('',#11948,#8733,#8734);
#7575=AXIS2_PLACEMENT_3D('',#12025,#8737,#8738);
#7576=AXIS2_PLACEMENT_3D('',#12103,#8742,#8743);
#7577=AXIS2_PLACEMENT_3D('',#12181,#8747,#8748);
#7578=AXIS2_PLACEMENT_3D('',#12259,#8752,#8753);
#7579=AXIS2_PLACEMENT_3D('',#12275,#8757,#8758);
#7580=AXIS2_PLACEMENT_3D('',#12599,#8770,#8771);
#7581=AXIS2_PLACEMENT_3D('',#12601,#8772,#8773);
#7582=AXIS2_PLACEMENT_3D('',#12603,#8775,#8776);
#7583=AXIS2_PLACEMENT_3D('',#12605,#8777,#8778);
#7584=AXIS2_PLACEMENT_3D('',#12607,#8780,#8781);
#7585=AXIS2_PLACEMENT_3D('',#12775,#8783,#8784);
#7586=AXIS2_PLACEMENT_3D('',#12776,#8785,#8786);
#7587=AXIS2_PLACEMENT_3D('',#12781,#8787,#8788);
#7588=AXIS2_PLACEMENT_3D('',#12853,#8790,#8791);
#7589=AXIS2_PLACEMENT_3D('',#12971,#8793,#8794);
#7590=AXIS2_PLACEMENT_3D('',#13016,#8795,#8796);
#7591=AXIS2_PLACEMENT_3D('',#13134,#8798,#8799);
#7592=AXIS2_PLACEMENT_3D('',#13179,#8800,#8801);
#7593=AXIS2_PLACEMENT_3D('',#13299,#8803,#8804);
#7594=AXIS2_PLACEMENT_3D('',#13304,#8805,#8806);
#7595=AXIS2_PLACEMENT_3D('',#13356,#8808,#8809);
#7596=AXIS2_PLACEMENT_3D('',#13357,#8810,#8811);
#7597=AXIS2_PLACEMENT_3D('',#13358,#8812,#8813);
#7598=AXIS2_PLACEMENT_3D('',#13359,#8814,#8815);
#7599=AXIS2_PLACEMENT_3D('',#13360,#8816,#8817);
#7600=AXIS2_PLACEMENT_3D('',#13361,#8818,#8819);
#7601=AXIS2_PLACEMENT_3D('',#13363,#8820,#8821);
#7602=AXIS2_PLACEMENT_3D('',#13364,#8822,#8823);
#7603=AXIS2_PLACEMENT_3D('',#13365,#8824,#8825);
#7604=AXIS2_PLACEMENT_3D('',#13366,#8826,#8827);
#7605=AXIS2_PLACEMENT_3D('',#13367,#8828,#8829);
#7606=AXIS2_PLACEMENT_3D('',#13368,#8830,#8831);
#7607=AXIS2_PLACEMENT_3D('',#13389,#8832,#8833);
#7608=AXIS2_PLACEMENT_3D('',#13391,#8834,#8835);
#7609=AXIS2_PLACEMENT_3D('',#13392,#8836,#8837);
#7610=AXIS2_PLACEMENT_3D('',#13393,#8838,#8839);
#7611=AXIS2_PLACEMENT_3D('',#13483,#8841,#8842);
#7612=AXIS2_PLACEMENT_3D('',#13484,#8843,#8844);
#7613=AXIS2_PLACEMENT_3D('',#13487,#8845,#8846);
#7614=AXIS2_PLACEMENT_3D('',#13489,#8847,#8848);
#7615=AXIS2_PLACEMENT_3D('',#13490,#8849,#8850);
#7616=AXIS2_PLACEMENT_3D('',#13491,#8851,#8852);
#7617=AXIS2_PLACEMENT_3D('',#13494,#8853,#8854);
#7618=AXIS2_PLACEMENT_3D('',#13496,#8855,#8856);
#7619=AXIS2_PLACEMENT_3D('',#13497,#8857,#8858);
#7620=AXIS2_PLACEMENT_3D('',#13498,#8859,#8860);
#7621=AXIS2_PLACEMENT_3D('',#13501,#8861,#8862);
#7622=AXIS2_PLACEMENT_3D('',#13503,#8863,#8864);
#7623=AXIS2_PLACEMENT_3D('',#13504,#8865,#8866);
#7624=AXIS2_PLACEMENT_3D('',#13505,#8867,#8868);
#7625=AXIS2_PLACEMENT_3D('',#13536,#8871,#8872);
#7626=AXIS2_PLACEMENT_3D('',#13539,#8873,#8874);
#7627=AXIS2_PLACEMENT_3D('',#13541,#8875,#8876);
#7628=AXIS2_PLACEMENT_3D('',#13542,#8877,#8878);
#7629=AXIS2_PLACEMENT_3D('',#13543,#8879,#8880);
#7630=AXIS2_PLACEMENT_3D('',#13723,#8883,#8884);
#7631=AXIS2_PLACEMENT_3D('',#13724,#8885,#8886);
#7632=AXIS2_PLACEMENT_3D('',#13741,#8887,#8888);
#8553=DIRECTION('axis',(0.,0.,1.));
#8554=DIRECTION('refdir',(1.,0.,0.));
#8555=DIRECTION('center_axis',(0.,0.,-1.));
#8556=DIRECTION('ref_axis',(1.,0.,0.));
#8557=DIRECTION('center_axis',(1.01338750660366E-31,-1.26069923670246E-19,
-1.));
#8558=DIRECTION('ref_axis',(1.,0.,0.));
#8559=DIRECTION('',(0.,0.,-1.));
#8560=DIRECTION('center_axis',(-1.01338750660366E-31,1.26069923670246E-19,
1.));
#8561=DIRECTION('ref_axis',(1.,0.,0.));
#8562=DIRECTION('center_axis',(0.,0.,-1.));
#8563=DIRECTION('ref_axis',(1.,0.,0.));
#8564=DIRECTION('center_axis',(1.01338750660366E-31,-1.26069923670246E-19,
-1.));
#8565=DIRECTION('ref_axis',(1.,0.,0.));
#8566=DIRECTION('',(0.,0.,-1.));
#8567=DIRECTION('center_axis',(-1.01338750660366E-31,1.26069923670246E-19,
1.));
#8568=DIRECTION('ref_axis',(1.,0.,0.));
#8569=DIRECTION('center_axis',(0.,0.,-1.));
#8570=DIRECTION('ref_axis',(1.,0.,0.));
#8571=DIRECTION('center_axis',(1.01338750660366E-31,-1.26069923670246E-19,
-1.));
#8572=DIRECTION('ref_axis',(1.,0.,0.));
#8573=DIRECTION('',(0.,0.,-1.));
#8574=DIRECTION('center_axis',(-1.01338750660366E-31,1.26069923670246E-19,
1.));
#8575=DIRECTION('ref_axis',(1.,0.,0.));
#8576=DIRECTION('center_axis',(0.,0.,-1.));
#8577=DIRECTION('ref_axis',(1.,0.,0.));
#8578=DIRECTION('center_axis',(1.01338750660366E-31,-1.26069923670246E-19,
-1.));
#8579=DIRECTION('ref_axis',(1.,0.,0.));
#8580=DIRECTION('',(0.,0.,-1.));
#8581=DIRECTION('center_axis',(-1.01338750660366E-31,1.26069923670246E-19,
1.));
#8582=DIRECTION('ref_axis',(1.,0.,0.));
#8583=DIRECTION('center_axis',(0.86602540378444,0.499999999999998,0.));
#8584=DIRECTION('ref_axis',(0.499999999999998,-0.86602540378444,0.));
#8585=DIRECTION('',(0.499999999999998,-0.86602540378444,1.09179756551649E-19));
#8586=DIRECTION('',(0.,0.,-1.));
#8587=DIRECTION('',(0.499999999999998,-0.86602540378444,0.));
#8588=DIRECTION('',(0.,0.,-1.));
#8589=DIRECTION('center_axis',(1.60246890531963E-16,1.,0.));
#8590=DIRECTION('ref_axis',(1.,-1.60246890531963E-16,0.));
#8591=DIRECTION('',(1.,-1.60246890531963E-16,1.01358952973624E-31));
#8592=DIRECTION('',(0.,0.,-1.));
#8593=DIRECTION('',(1.,-1.60246890531963E-16,0.));
#8594=DIRECTION('center_axis',(-0.86602540378444,0.499999999999998,0.));
#8595=DIRECTION('ref_axis',(0.499999999999998,0.86602540378444,0.));
#8596=DIRECTION('',(0.499999999999998,0.86602540378444,-1.09179756551548E-19));
#8597=DIRECTION('',(0.,0.,-1.));
#8598=DIRECTION('',(0.499999999999998,0.86602540378444,0.));
#8599=DIRECTION('center_axis',(-0.86602540378444,-0.499999999999998,0.));
#8600=DIRECTION('ref_axis',(-0.499999999999998,0.86602540378444,0.));
#8601=DIRECTION('',(-0.499999999999998,0.86602540378444,-1.09179756551649E-19));
#8602=DIRECTION('',(0.,0.,-1.));
#8603=DIRECTION('',(-0.499999999999998,0.86602540378444,0.));
#8604=DIRECTION('center_axis',(-1.60246890531963E-16,-1.,0.));
#8605=DIRECTION('ref_axis',(-1.,1.60246890531963E-16,0.));
#8606=DIRECTION('',(-1.,1.60246890531963E-16,-1.01358952973624E-31));
#8607=DIRECTION('',(0.,0.,-1.));
#8608=DIRECTION('',(-1.,1.60246890531963E-16,0.));
#8609=DIRECTION('center_axis',(0.86602540378444,-0.499999999999998,0.));
#8610=DIRECTION('ref_axis',(-0.499999999999998,-0.86602540378444,0.));
#8611=DIRECTION('',(-0.499999999999998,-0.86602540378444,1.09179756551548E-19));
#8612=DIRECTION('',(-0.499999999999998,-0.86602540378444,0.));
#8613=DIRECTION('center_axis',(0.,0.,-1.));
#8614=DIRECTION('ref_axis',(-1.,0.,0.));
#8615=DIRECTION('center_axis',(0.,0.,1.));
#8616=DIRECTION('ref_axis',(1.,0.,0.));
#8617=DIRECTION('center_axis',(0.866025403784439,0.5,0.));
#8618=DIRECTION('ref_axis',(0.5,-0.866025403784439,0.));
#8619=DIRECTION('',(0.5,-0.866025403784439,1.09179756551649E-19));
#8620=DIRECTION('',(0.,0.,-1.));
#8621=DIRECTION('',(0.5,-0.866025403784439,0.));
#8622=DIRECTION('',(0.,0.,-1.));
#8623=DIRECTION('center_axis',(1.60246890531964E-16,1.,0.));
#8624=DIRECTION('ref_axis',(1.,-1.60246890531964E-16,0.));
#8625=DIRECTION('',(1.,-1.60246890531964E-16,1.01358952973624E-31));
#8626=DIRECTION('',(0.,0.,-1.));
#8627=DIRECTION('',(1.,-1.60246890531964E-16,0.));
#8628=DIRECTION('center_axis',(-0.866025403784438,0.5,0.));
#8629=DIRECTION('ref_axis',(0.5,0.866025403784438,0.));
#8630=DIRECTION('',(0.5,0.866025403784438,-1.09179756551547E-19));
#8631=DIRECTION('',(0.,0.,-1.));
#8632=DIRECTION('',(0.5,0.866025403784438,0.));
#8633=DIRECTION('center_axis',(-0.866025403784439,-0.499999999999999,0.));
#8634=DIRECTION('ref_axis',(-0.499999999999999,0.866025403784439,0.));
#8635=DIRECTION('',(-0.499999999999999,0.866025403784439,-1.09179756551649E-19));
#8636=DIRECTION('',(0.,0.,-1.));
#8637=DIRECTION('',(-0.499999999999999,0.866025403784439,0.));
#8638=DIRECTION('center_axis',(-1.60246890531964E-16,-1.,0.));
#8639=DIRECTION('ref_axis',(-1.,1.60246890531964E-16,0.));
#8640=DIRECTION('',(-1.,1.60246890531964E-16,-1.01358952973624E-31));
#8641=DIRECTION('',(0.,0.,-1.));
#8642=DIRECTION('',(-1.,1.60246890531964E-16,0.));
#8643=DIRECTION('center_axis',(0.866025403784439,-0.5,0.));
#8644=DIRECTION('ref_axis',(-0.5,-0.866025403784439,0.));
#8645=DIRECTION('',(-0.5,-0.866025403784439,1.09179756551547E-19));
#8646=DIRECTION('',(-0.5,-0.866025403784439,0.));
#8647=DIRECTION('center_axis',(0.,0.,-1.));
#8648=DIRECTION('ref_axis',(-1.,0.,0.));
#8649=DIRECTION('center_axis',(0.,0.,1.));
#8650=DIRECTION('ref_axis',(1.,0.,0.));
#8651=DIRECTION('center_axis',(0.,0.,-1.));
#8652=DIRECTION('ref_axis',(1.,0.,0.));
#8653=DIRECTION('',(0.,0.,-1.));
#8654=DIRECTION('center_axis',(0.,0.,1.));
#8655=DIRECTION('ref_axis',(1.,0.,0.));
#8656=DIRECTION('center_axis',(0.,0.,-1.));
#8657=DIRECTION('ref_axis',(1.,0.,0.));
#8658=DIRECTION('',(0.,0.,-1.));
#8659=DIRECTION('center_axis',(0.,0.,1.));
#8660=DIRECTION('ref_axis',(1.,0.,0.));
#8661=DIRECTION('center_axis',(0.,-1.,0.));
#8662=DIRECTION('ref_axis',(-1.,0.,0.));
#8663=DIRECTION('',(0.0523359562429438,0.,0.998629534754574));
#8664=DIRECTION('',(1.,0.,0.));
#8665=DIRECTION('',(-0.0523359562429438,0.,-0.998629534754574));
#8666=DIRECTION('',(1.,0.,0.));
#8667=DIRECTION('center_axis',(0.,-1.,0.));
#8668=DIRECTION('ref_axis',(-1.,0.,0.));
#8669=DIRECTION('',(0.,0.,-1.));
#8670=DIRECTION('',(1.,0.,0.));
#8671=DIRECTION('',(0.,0.,1.));
#8672=DIRECTION('',(1.,0.,0.));
#8673=DIRECTION('center_axis',(0.,-1.,0.));
#8674=DIRECTION('ref_axis',(-1.,0.,0.));
#8675=DIRECTION('',(0.,0.,-1.));
#8676=DIRECTION('',(1.,0.,0.));
#8677=DIRECTION('',(0.,0.,1.));
#8678=DIRECTION('',(1.,0.,0.));
#8679=DIRECTION('center_axis',(0.,-1.,0.));
#8680=DIRECTION('ref_axis',(-1.,0.,0.));
#8681=DIRECTION('',(0.,0.,-1.));
#8682=DIRECTION('',(1.,0.,0.));
#8683=DIRECTION('',(0.,0.,1.));
#8684=DIRECTION('',(1.,0.,0.));
#8685=DIRECTION('center_axis',(0.,1.,0.));
#8686=DIRECTION('ref_axis',(1.,0.,0.));
#8687=DIRECTION('',(-0.0523359562429438,0.,-0.998629534754574));
#8688=DIRECTION('',(-1.,0.,0.));
#8689=DIRECTION('',(0.0523359562429438,0.,0.998629534754574));
#8690=DIRECTION('',(-1.,0.,0.));
#8691=DIRECTION('center_axis',(0.,1.,0.));
#8692=DIRECTION('ref_axis',(1.,0.,0.));
#8693=DIRECTION('',(0.,0.,1.));
#8694=DIRECTION('',(-1.,0.,0.));
#8695=DIRECTION('',(0.,0.,-1.));
#8696=DIRECTION('',(-1.,0.,0.));
#8697=DIRECTION('center_axis',(0.,1.,0.));
#8698=DIRECTION('ref_axis',(1.,0.,0.));
#8699=DIRECTION('',(0.,0.,1.));
#8700=DIRECTION('',(-1.,0.,0.));
#8701=DIRECTION('',(0.,0.,-1.));
#8702=DIRECTION('',(-1.,0.,0.));
#8703=DIRECTION('center_axis',(0.,0.,1.));
#8704=DIRECTION('ref_axis',(1.,0.,0.));
#8705=DIRECTION('center_axis',(0.,0.,1.));
#8706=DIRECTION('ref_axis',(1.,0.,0.));
#8707=DIRECTION('center_axis',(0.,0.,1.));
#8708=DIRECTION('ref_axis',(1.,0.,0.));
#8709=DIRECTION('center_axis',(0.,0.,1.));
#8710=DIRECTION('ref_axis',(1.,0.,0.));
#8711=DIRECTION('center_axis',(0.,0.,1.));
#8712=DIRECTION('ref_axis',(1.,0.,0.));
#8713=DIRECTION('',(0.,1.,0.));
#8714=DIRECTION('',(0.,-1.,0.));
#8715=DIRECTION('center_axis',(0.,0.,1.));
#8716=DIRECTION('ref_axis',(1.,0.,0.));
#8717=DIRECTION('',(0.,-1.,0.));
#8718=DIRECTION('',(0.,1.,0.));
#8719=DIRECTION('center_axis',(0.,0.,1.));
#8720=DIRECTION('ref_axis',(1.,0.,0.));
#8721=DIRECTION('',(0.,-1.,0.));
#8722=DIRECTION('',(0.,1.,0.));
#8723=DIRECTION('center_axis',(0.,0.,1.));
#8724=DIRECTION('ref_axis',(1.,0.,0.));
#8725=DIRECTION('',(0.,-1.,0.));
#8726=DIRECTION('',(-1.,0.,0.));
#8727=DIRECTION('',(0.,1.,0.));
#8728=DIRECTION('center_axis',(0.,1.,0.));
#8729=DIRECTION('ref_axis',(1.,0.,0.));
#8730=DIRECTION('',(0.,0.,1.));
#8731=DIRECTION('',(-1.,0.,0.));
#8732=DIRECTION('',(0.,0.,-1.));
#8733=DIRECTION('center_axis',(-1.,0.,0.));
#8734=DIRECTION('ref_axis',(0.,-1.,0.));
#8735=DIRECTION('',(0.,-1.,0.));
#8736=DIRECTION('',(0.,-1.,1.26069923670246E-19));
#8737=DIRECTION('center_axis',(1.,0.,0.));
#8738=DIRECTION('ref_axis',(0.,1.,0.));
#8739=DIRECTION('',(0.,1.,0.));
#8740=DIRECTION('',(0.,1.,-1.26069923670246E-19));
#8741=DIRECTION('',(0.,1.,0.));
#8742=DIRECTION('center_axis',(1.,0.,0.));
#8743=DIRECTION('ref_axis',(0.,1.,0.));
#8744=DIRECTION('',(0.,1.,0.));
#8745=DIRECTION('',(0.,1.,-1.26069923670246E-19));
#8746=DIRECTION('',(0.,1.,0.));
#8747=DIRECTION('center_axis',(1.,0.,0.));
#8748=DIRECTION('ref_axis',(0.,1.,0.));
#8749=DIRECTION('',(0.,1.,0.));
#8750=DIRECTION('',(0.,1.,-1.26069923670246E-19));
#8751=DIRECTION('',(0.,1.,0.));
#8752=DIRECTION('center_axis',(0.998629534754574,0.,-0.0523359562429438));
#8753=DIRECTION('ref_axis',(-0.0523359562429438,0.,-0.998629534754574));
#8754=DIRECTION('',(0.,-1.,0.));
#8755=DIRECTION('',(6.6070447339401E-21,-1.,1.26069923670246E-19));
#8756=DIRECTION('',(0.,-1.,0.));
#8757=DIRECTION('center_axis',(0.,0.,1.));
#8758=DIRECTION('ref_axis',(1.,0.,0.));
#8759=DIRECTION('',(0.,-1.,0.));
#8760=DIRECTION('',(0.,-1.,0.));
#8761=DIRECTION('',(0.,-1.,0.));
#8762=DIRECTION('',(0.,1.,0.));
#8763=DIRECTION('',(0.,-1.,0.));
#8764=DIRECTION('',(0.,1.,0.));
#8765=DIRECTION('',(0.,-1.,0.));
#8766=DIRECTION('',(0.,-1.,0.));
#8767=DIRECTION('',(0.,-1.,0.));
#8768=DIRECTION('',(0.,1.,0.));
#8769=DIRECTION('',(0.,1.,0.));
#8770=DIRECTION('center_axis',(0.,0.,1.));
#8771=DIRECTION('ref_axis',(1.,0.,0.));
#8772=DIRECTION('center_axis',(-1.01338750660366E-31,1.26069923670246E-19,
1.));
#8773=DIRECTION('ref_axis',(1.,0.,0.));
#8774=DIRECTION('',(0.,0.,-1.));
#8775=DIRECTION('center_axis',(0.,0.,1.));
#8776=DIRECTION('ref_axis',(1.,0.,0.));
#8777=DIRECTION('center_axis',(-1.01338750660366E-31,1.26069923670246E-19,
1.));
#8778=DIRECTION('ref_axis',(1.,0.,0.));
#8779=DIRECTION('',(0.,0.,-1.));
#8780=DIRECTION('center_axis',(1.,0.,0.));
#8781=DIRECTION('ref_axis',(0.,1.,0.));
#8782=DIRECTION('',(0.,1.,-1.26069923670246E-19));
#8783=DIRECTION('center_axis',(0.995216631131787,0.0976926666577189,1.18580395612125E-14));
#8784=DIRECTION('ref_axis',(0.0975341006448478,-0.993601284365854,0.0569524970297685));
#8785=DIRECTION('center_axis',(-1.01338750660366E-31,1.26069923670246E-19,
1.));
#8786=DIRECTION('ref_axis',(1.,0.,1.01338750660366E-31));
#8787=DIRECTION('center_axis',(-1.01338750660366E-31,1.26069923670246E-19,
1.));
#8788=DIRECTION('ref_axis',(1.,0.,1.01338750660366E-31));
#8789=DIRECTION('',(-6.60704473394009E-21,-1.,1.26069923670246E-19));
#8790=DIRECTION('center_axis',(-1.,0.,0.));
#8791=DIRECTION('ref_axis',(0.,-1.,0.));
#8792=DIRECTION('',(0.,-1.,1.26069923670246E-19));
#8793=DIRECTION('center_axis',(-1.01338750660366E-31,1.26069923670246E-19,
1.));
#8794=DIRECTION('ref_axis',(1.,0.,1.01338750660366E-31));
#8795=DIRECTION('center_axis',(-1.,0.,0.));
#8796=DIRECTION('ref_axis',(0.,-1.,0.));
#8797=DIRECTION('',(0.,-1.,1.26069923670246E-19));
#8798=DIRECTION('center_axis',(-1.01338750660366E-31,1.26069923670246E-19,
1.));
#8799=DIRECTION('ref_axis',(1.,0.,1.01338750660366E-31));
#8800=DIRECTION('center_axis',(-1.,0.,0.));
#8801=DIRECTION('ref_axis',(0.,-1.,0.));
#8802=DIRECTION('',(0.,-1.,1.26069923670246E-19));
#8803=DIRECTION('center_axis',(-0.982258063247475,0.187534256031586,1.45403402392141E-15));
#8804=DIRECTION('ref_axis',(1.48029736616688E-15,0.,1.));
#8805=DIRECTION('center_axis',(-1.01338750660366E-31,1.26069923670246E-19,
1.));
#8806=DIRECTION('ref_axis',(1.,0.,1.01338750660366E-31));
#8807=DIRECTION('',(-6.6070447339401E-21,1.,-1.26069923670246E-19));
#8808=DIRECTION('center_axis',(-0.982258063247479,-0.187534256031562,9.14061384143289E-15));
#8809=DIRECTION('ref_axis',(-0.187187393251729,0.980441281772238,0.0607928680392112));
#8810=DIRECTION('center_axis',(-0.45173408531537,0.373496730537872,-0.810207694632559));
#8811=DIRECTION('ref_axis',(-0.624418441188311,0.516273298501642,0.586142893463867));
#8812=DIRECTION('center_axis',(-2.96465769266614E-15,1.,0.));
#8813=DIRECTION('ref_axis',(0.,0.,1.));
#8814=DIRECTION('center_axis',(0.0522655346583812,-0.0518587053130894,0.997285810873755));
#8815=DIRECTION('ref_axis',(-0.998629534754574,0.,0.0523359562429445));
#8816=DIRECTION('center_axis',(0.377681861983732,-0.843372107574977,0.38220400219391));
#8817=DIRECTION('ref_axis',(0.592794689304902,0.537329962094562,0.599892463836113));
#8818=DIRECTION('center_axis',(0.995216631131786,-0.0976926666577302,0.));
#8819=DIRECTION('ref_axis',(0.,0.,1.));
#8820=DIRECTION('center_axis',(-0.0522650609395843,-0.052032719242908,0.997276771780618));
#8821=DIRECTION('ref_axis',(0.0975341006448596,0.993601284365853,0.0569524970297681));
#8822=DIRECTION('center_axis',(1.55158195278682E-16,1.,-2.96059473233375E-15));
#8823=DIRECTION('ref_axis',(0.998629534754574,0.,0.0523359562429438));
#8824=DIRECTION('center_axis',(-0.45173408531537,-0.373496730537869,-0.810207694632561));
#8825=DIRECTION('ref_axis',(-0.624418441188315,-0.516273298501641,0.586142893463864));
#8826=DIRECTION('center_axis',(0.0522655346583823,0.0518587053130918,0.997285810873755));
#8827=DIRECTION('ref_axis',(-0.187187393251729,-0.980441281772238,0.0607928680392122));
#8828=DIRECTION('center_axis',(-2.71526841737693E-16,-1.,-5.18104078158406E-15));
#8829=DIRECTION('ref_axis',(-0.998629534754574,0.,0.0523359562429439));
#8830=DIRECTION('center_axis',(-6.6070447339401E-21,1.,-1.26069923670246E-19));
#8831=DIRECTION('ref_axis',(-0.688354575693753,0.,0.725374371012289));
#8832=DIRECTION('center_axis',(-0.377681861983722,-0.843372107574983,-0.382204002193908));
#8833=DIRECTION('ref_axis',(0.592794689304909,-0.537329962094554,0.599892463836112));
#8834=DIRECTION('center_axis',(-0.0522650609395818,0.0520327192429072,0.997276771780618));
#8835=DIRECTION('ref_axis',(0.998629534754574,0.,0.0523359562429431));
#8836=DIRECTION('center_axis',(2.96465769266612E-15,-1.,0.));
#8837=DIRECTION('ref_axis',(0.,0.,1.));
#8838=DIRECTION('center_axis',(-6.60704473394009E-21,-1.,1.26069923670246E-19));
#8839=DIRECTION('ref_axis',(0.688354575693758,0.,0.725374371012284));
#8840=DIRECTION('',(6.60704473394009E-21,1.,-1.26069923670246E-19));
#8841=DIRECTION('center_axis',(-0.998629534754574,0.,-0.0523359562429438));
#8842=DIRECTION('ref_axis',(-0.0523359562429438,0.,0.998629534754574));
#8843=DIRECTION('center_axis',(-0.45173408531537,0.373496730537872,-0.81020769463256));
#8844=DIRECTION('ref_axis',(-0.624418441188311,0.516273298501643,0.586142893463866));
#8845=DIRECTION('center_axis',(-2.96465769266614E-15,1.,0.));
#8846=DIRECTION('ref_axis',(0.,0.,1.));
#8847=DIRECTION('center_axis',(-0.982258063247479,-0.187534256031562,9.14061384143289E-15));
#8848=DIRECTION('ref_axis',(-0.187187393251729,0.980441281772238,0.0607928680392111));
#8849=DIRECTION('center_axis',(0.0522655346583812,-0.0518587053130894,0.997285810873755));
#8850=DIRECTION('ref_axis',(-0.998629534754574,0.,0.0523359562429445));
#8851=DIRECTION('center_axis',(0.377681861983731,-0.843372107574978,0.38220400219391));
#8852=DIRECTION('ref_axis',(0.592794689304906,0.537329962094559,0.599892463836111));
#8853=DIRECTION('center_axis',(0.995216631131786,-0.0976926666577302,0.));
#8854=DIRECTION('ref_axis',(0.,0.,1.));
#8855=DIRECTION('center_axis',(1.55158195278682E-16,1.,-2.96059473233375E-15));
#8856=DIRECTION('ref_axis',(0.998629534754574,0.,0.0523359562429438));
#8857=DIRECTION('center_axis',(-0.0522650609395843,-0.052032719242908,0.997276771780618));
#8858=DIRECTION('ref_axis',(0.0975341006448596,0.993601284365853,0.0569524970297681));
#8859=DIRECTION('center_axis',(-0.45173408531537,-0.373496730537868,-0.810207694632561));
#8860=DIRECTION('ref_axis',(-0.624418441188315,-0.516273298501641,0.586142893463864));
#8861=DIRECTION('center_axis',(-0.982258063247475,0.187534256031586,1.45403402392141E-15));
#8862=DIRECTION('ref_axis',(1.48029736616688E-15,0.,1.));
#8863=DIRECTION('center_axis',(-2.71526841737693E-16,-1.,-5.18104078158406E-15));
#8864=DIRECTION('ref_axis',(-0.998629534754574,0.,0.0523359562429439));
#8865=DIRECTION('center_axis',(0.0522655346583823,0.0518587053130918,0.997285810873755));
#8866=DIRECTION('ref_axis',(-0.187187393251729,-0.980441281772238,0.0607928680392122));
#8867=DIRECTION('center_axis',(-6.6070447339401E-21,1.,-1.26069923670246E-19));
#8868=DIRECTION('ref_axis',(-0.688354575693753,0.,0.725374371012289));
#8869=DIRECTION('',(6.6070447339401E-21,-1.,1.26069923670246E-19));
#8870=DIRECTION('',(-6.6070447339401E-21,1.,-1.26069923670246E-19));
#8871=DIRECTION('center_axis',(-0.377681861983727,-0.843372107574981,-0.382204002193907));
#8872=DIRECTION('ref_axis',(0.592794689304909,-0.537329962094554,0.599892463836112));
#8873=DIRECTION('center_axis',(-0.0522650609395818,0.0520327192429072,0.997276771780618));
#8874=DIRECTION('ref_axis',(0.998629534754574,0.,0.0523359562429431));
#8875=DIRECTION('center_axis',(2.96465769266612E-15,-1.,0.));
#8876=DIRECTION('ref_axis',(0.,0.,1.));
#8877=DIRECTION('center_axis',(0.995216631131787,0.0976926666577189,1.18580395612125E-14));
#8878=DIRECTION('ref_axis',(0.0975341006448478,-0.993601284365854,0.0569524970297685));
#8879=DIRECTION('center_axis',(-6.60704473394009E-21,-1.,1.26069923670246E-19));
#8880=DIRECTION('ref_axis',(0.688354575693758,0.,0.725374371012284));
#8881=DIRECTION('',(6.60704473394009E-21,1.,-1.26069923670246E-19));
#8882=DIRECTION('',(-6.60704473394009E-21,-1.,1.26069923670246E-19));
#8883=DIRECTION('center_axis',(0.998629534754574,0.,-0.0523359562429438));
#8884=DIRECTION('ref_axis',(-0.0523359562429438,0.,-0.998629534754574));
#8885=DIRECTION('center_axis',(-1.01338750660366E-31,1.26069923670246E-19,
1.));
#8886=DIRECTION('ref_axis',(1.,0.,1.01338750660366E-31));
#8887=DIRECTION('center_axis',(-0.998629534754574,0.,-0.0523359562429438));
#8888=DIRECTION('ref_axis',(-0.0523359562429438,0.,0.998629534754574));
#11747=CARTESIAN_POINT('',(0.,0.,0.));
#11748=CARTESIAN_POINT('Origin',(9.,-1.,0.8));
#11749=CARTESIAN_POINT('',(8.85,-1.,0.9));
#11750=CARTESIAN_POINT('Origin',(9.,-1.,0.9));
#11751=CARTESIAN_POINT('',(8.85,-1.,0.7));
#11752=CARTESIAN_POINT('',(8.85,-1.,0.8));
#11753=CARTESIAN_POINT('Origin',(9.,-1.,0.7));
#11754=CARTESIAN_POINT('Origin',(3.,-1.,0.8));
#11755=CARTESIAN_POINT('',(2.85,-1.,0.9));
#11756=CARTESIAN_POINT('Origin',(3.,-1.,0.9));
#11757=CARTESIAN_POINT('',(2.85,-1.,0.7));
#11758=CARTESIAN_POINT('',(2.85,-1.,0.8));
#11759=CARTESIAN_POINT('Origin',(3.,-1.,0.7));
#11760=CARTESIAN_POINT('Origin',(3.,1.,0.8));
#11761=CARTESIAN_POINT('',(2.85,1.,0.9));
#11762=CARTESIAN_POINT('Origin',(3.,1.,0.9));
#11763=CARTESIAN_POINT('',(2.85,1.,0.7));
#11764=CARTESIAN_POINT('',(2.85,1.,0.8));
#11765=CARTESIAN_POINT('Origin',(3.,1.,0.7));
#11766=CARTESIAN_POINT('Origin',(9.,1.,0.8));
#11767=CARTESIAN_POINT('',(8.85,1.,0.9));
#11768=CARTESIAN_POINT('Origin',(9.,1.,0.9));
#11769=CARTESIAN_POINT('',(8.85,1.,0.7));
#11770=CARTESIAN_POINT('',(8.85,1.,0.8));
#11771=CARTESIAN_POINT('Origin',(9.,1.,0.7));
#11772=CARTESIAN_POINT('Origin',(10.1732050807569,0.3,0.9));
#11773=CARTESIAN_POINT('',(10.1732050807569,0.3,0.9));
#11774=CARTESIAN_POINT('',(10.3464101615138,0.,0.9));
#11775=CARTESIAN_POINT('',(9.72652155859676,1.07367855528516,0.9));
#11776=CARTESIAN_POINT('',(10.1732050807569,0.3,0.6));
#11777=CARTESIAN_POINT('',(10.1732050807569,0.3,0.9));
#11778=CARTESIAN_POINT('',(10.3464101615138,0.,0.6));
#11779=CARTESIAN_POINT('',(10.3464101615138,0.,0.6));
#11780=CARTESIAN_POINT('',(10.3464101615138,0.,0.9));
#11781=CARTESIAN_POINT('Origin',(9.82679491924311,0.3,0.9));
#11782=CARTESIAN_POINT('',(9.82679491924311,0.3,0.9));
#11783=CARTESIAN_POINT('',(7.95345829022414,0.3,0.9));
#11784=CARTESIAN_POINT('',(9.82679491924311,0.3,0.6));
#11785=CARTESIAN_POINT('',(9.82679491924311,0.3,0.9));
#11786=CARTESIAN_POINT('',(10.1732050807569,0.3,0.6));
#11787=CARTESIAN_POINT('Origin',(9.65358983848622,5.55111512312578E-17,
0.9));
#11788=CARTESIAN_POINT('',(9.65358983848622,4.24230095489963E-17,0.9));
#11789=CARTESIAN_POINT('',(9.2069063163261,-0.773678555285165,0.9));
#11790=CARTESIAN_POINT('',(9.65358983848622,5.55111512312578E-17,0.6));
#11791=CARTESIAN_POINT('',(9.65358983848622,4.24230095489963E-17,0.9));
#11792=CARTESIAN_POINT('',(9.82679491924311,0.3,0.6));
#11793=CARTESIAN_POINT('Origin',(9.82679491924311,-0.3,0.9));
#11794=CARTESIAN_POINT('',(9.82679491924311,-0.3,0.9));
#11795=CARTESIAN_POINT('',(9.29350885670454,0.623678555285165,0.9));
#11796=CARTESIAN_POINT('',(9.82679491924311,-0.3,0.6));
#11797=CARTESIAN_POINT('',(9.82679491924311,-0.3,0.9));
#11798=CARTESIAN_POINT('',(9.65358983848622,4.24230095489963E-17,0.6));
#11799=CARTESIAN_POINT('Origin',(10.1732050807569,-0.3,0.9));
#11800=CARTESIAN_POINT('',(10.1732050807569,-0.3,0.9));
#11801=CARTESIAN_POINT('',(8.12666337098103,-0.3,0.9));
#11802=CARTESIAN_POINT('',(10.1732050807569,-0.3,0.6));
#11803=CARTESIAN_POINT('',(10.1732050807569,-0.3,0.9));
#11804=CARTESIAN_POINT('',(9.82679491924311,-0.3,0.6));
#11805=CARTESIAN_POINT('Origin',(10.3464101615138,0.,0.9));
#11806=CARTESIAN_POINT('',(9.8131240989752,-0.923678555285165,0.9));
#11807=CARTESIAN_POINT('',(10.1732050807569,-0.3,0.6));
#11808=CARTESIAN_POINT('Origin',(10.,5.55111512312578E-17,0.6));
#11809=CARTESIAN_POINT('',(9.83,-2.0818995585505E-17,0.6));
#11810=CARTESIAN_POINT('Origin',(10.,0.,0.6));
#11811=CARTESIAN_POINT('Origin',(2.17320508075689,0.3,0.9));
#11812=CARTESIAN_POINT('',(2.17320508075689,0.3,0.9));
#11813=CARTESIAN_POINT('',(2.34641016151378,0.,0.9));
#11814=CARTESIAN_POINT('',(2.72652155859676,-0.65837225228371,0.9));
#11815=CARTESIAN_POINT('',(2.17320508075689,0.3,0.6));
#11816=CARTESIAN_POINT('',(2.17320508075689,0.3,0.9));
#11817=CARTESIAN_POINT('',(2.34641016151378,0.,0.6));
#11818=CARTESIAN_POINT('',(2.34641016151378,0.,0.6));
#11819=CARTESIAN_POINT('',(2.34641016151378,0.,0.9));
#11820=CARTESIAN_POINT('Origin',(1.82679491924311,0.3,0.9));
#11821=CARTESIAN_POINT('',(1.82679491924311,0.3,0.9));
#11822=CARTESIAN_POINT('',(3.95345829022414,0.3,0.9));
#11823=CARTESIAN_POINT('',(1.82679491924311,0.3,0.6));
#11824=CARTESIAN_POINT('',(1.82679491924311,0.3,0.9));
#11825=CARTESIAN_POINT('',(2.17320508075689,0.3,0.6));
#11826=CARTESIAN_POINT('Origin',(1.65358983848622,5.55111512312578E-17,
0.9));
#11827=CARTESIAN_POINT('',(1.65358983848622,4.24230095489963E-17,0.9));
#11828=CARTESIAN_POINT('',(2.20690631632609,0.958372252283711,0.9));
#11829=CARTESIAN_POINT('',(1.65358983848622,5.55111512312578E-17,0.6));
#11830=CARTESIAN_POINT('',(1.65358983848622,4.24230095489963E-17,0.9));
#11831=CARTESIAN_POINT('',(1.82679491924311,0.3,0.6));
#11832=CARTESIAN_POINT('Origin',(1.82679491924311,-0.3,0.9));
#11833=CARTESIAN_POINT('',(1.82679491924311,-0.3,0.9));
#11834=CARTESIAN_POINT('',(2.29350885670453,-1.10837225228371,0.9));
#11835=CARTESIAN_POINT('',(1.82679491924311,-0.3,0.6));
#11836=CARTESIAN_POINT('',(1.82679491924311,-0.3,0.9));
#11837=CARTESIAN_POINT('',(1.65358983848622,4.24230095489963E-17,0.6));
#11838=CARTESIAN_POINT('Origin',(2.17320508075689,-0.3,0.9));
#11839=CARTESIAN_POINT('',(2.17320508075689,-0.3,0.9));
#11840=CARTESIAN_POINT('',(4.12666337098103,-0.3,0.9));
#11841=CARTESIAN_POINT('',(2.17320508075689,-0.3,0.6));
#11842=CARTESIAN_POINT('',(2.17320508075689,-0.3,0.9));
#11843=CARTESIAN_POINT('',(1.82679491924311,-0.3,0.6));
#11844=CARTESIAN_POINT('Origin',(2.34641016151378,0.,0.9));
#11845=CARTESIAN_POINT('',(2.8131240989752,0.80837225228371,0.9));
#11846=CARTESIAN_POINT('',(2.17320508075689,-0.3,0.6));
#11847=CARTESIAN_POINT('Origin',(2.,5.55111512312578E-17,0.6));
#11848=CARTESIAN_POINT('',(1.83,-2.0818995585505E-17,0.6));
#11849=CARTESIAN_POINT('Origin',(2.,0.,0.6));
#11850=CARTESIAN_POINT('Origin',(2.,0.,0.45));
#11851=CARTESIAN_POINT('',(1.83,-2.0818995585505E-17,0.32));
#11852=CARTESIAN_POINT('',(1.83,2.0818995585505E-17,0.45));
#11853=CARTESIAN_POINT('Origin',(2.,0.,0.32));
#11854=CARTESIAN_POINT('Origin',(10.,0.,0.45));
#11855=CARTESIAN_POINT('',(9.83,-2.0818995585505E-17,0.32));
#11856=CARTESIAN_POINT('',(9.83,2.0818995585505E-17,0.45));
#11857=CARTESIAN_POINT('Origin',(10.,0.,0.32));
#11858=CARTESIAN_POINT('Origin',(11.2,-0.62,0.32));
#11859=CARTESIAN_POINT('',(0.200274469199584,-0.62,0.));
#11860=CARTESIAN_POINT('',(0.217044958570157,-0.62,0.32));
#11861=CARTESIAN_POINT('',(0.223426876981161,-0.62,0.441774257530303));
#11862=CARTESIAN_POINT('',(0.,-0.62,0.));
#11863=CARTESIAN_POINT('',(8.63987299740311,-0.62,0.));
#11864=CARTESIAN_POINT('',(0.0167704893705732,-0.62,0.32));
#11865=CARTESIAN_POINT('',(0.0237009700302462,-0.62,0.452241448778892));
#11866=CARTESIAN_POINT('',(-0.1,-0.62,0.32));
#11867=CARTESIAN_POINT('Origin',(11.2,-0.62,0.32));
#11868=CARTESIAN_POINT('',(0.9,-0.62,0.32));
#11869=CARTESIAN_POINT('',(0.9,-0.62,0.));
#11870=CARTESIAN_POINT('',(0.9,-0.62,0.16));
#11871=CARTESIAN_POINT('',(1.1,-0.62,0.32));
#11872=CARTESIAN_POINT('',(-0.1,-0.62,0.32));
#11873=CARTESIAN_POINT('',(1.1,-0.62,0.));
#11874=CARTESIAN_POINT('',(1.1,-0.62,0.16));
#11875=CARTESIAN_POINT('',(8.63987299740311,-0.62,0.));
#11876=CARTESIAN_POINT('Origin',(11.2,-0.62,0.32));
#11877=CARTESIAN_POINT('',(3.9,-0.62,0.32));
#11878=CARTESIAN_POINT('',(3.9,-0.62,0.));
#11879=CARTESIAN_POINT('',(3.9,-0.62,0.16));
#11880=CARTESIAN_POINT('',(4.1,-0.62,0.32));
#11881=CARTESIAN_POINT('',(-0.1,-0.62,0.32));
#11882=CARTESIAN_POINT('',(4.1,-0.62,0.));
#11883=CARTESIAN_POINT('',(4.1,-0.62,0.16));
#11884=CARTESIAN_POINT('',(8.63987299740311,-0.62,0.));
#11885=CARTESIAN_POINT('Origin',(11.2,-0.62,0.32));
#11886=CARTESIAN_POINT('',(7.9,-0.62,0.32));
#11887=CARTESIAN_POINT('',(7.9,-0.62,0.));
#11888=CARTESIAN_POINT('',(7.9,-0.62,0.16));
#11889=CARTESIAN_POINT('',(8.1,-0.62,0.32));
#11890=CARTESIAN_POINT('',(-0.1,-0.62,0.32));
#11891=CARTESIAN_POINT('',(8.1,-0.62,0.));
#11892=CARTESIAN_POINT('',(8.1,-0.62,0.16));
#11893=CARTESIAN_POINT('',(8.63987299740311,-0.62,0.));
#11894=CARTESIAN_POINT('Origin',(-0.0999999999999996,0.62,0.32));
#11895=CARTESIAN_POINT('',(0.217044958570158,0.62,0.32));
#11896=CARTESIAN_POINT('',(0.200274469199586,0.62,0.));
#11897=CARTESIAN_POINT('',(0.207951231396534,0.62,0.146481348799182));
#11898=CARTESIAN_POINT('',(0.0167704893705736,0.62,0.32));
#11899=CARTESIAN_POINT('',(11.2,0.62,0.32));
#11900=CARTESIAN_POINT('',(0.,0.62,0.));
#11901=CARTESIAN_POINT('',(0.00822532444561912,0.62,0.156948540047771));
#11902=CARTESIAN_POINT('',(2.98987299740311,0.62,0.));
#11903=CARTESIAN_POINT('Origin',(-0.0999999999999996,0.62,0.32));
#11904=CARTESIAN_POINT('',(0.9,0.62,0.));
#11905=CARTESIAN_POINT('',(0.9,0.62,0.32));
#11906=CARTESIAN_POINT('',(0.9,0.62,0.16));
#11907=CARTESIAN_POINT('',(1.1,0.62,0.));
#11908=CARTESIAN_POINT('',(2.98987299740311,0.62,0.));
#11909=CARTESIAN_POINT('',(1.1,0.62,0.32));
#11910=CARTESIAN_POINT('',(1.1,0.62,0.16));
#11911=CARTESIAN_POINT('',(11.2,0.62,0.32));
#11912=CARTESIAN_POINT('Origin',(-0.0999999999999996,0.62,0.32));
#11913=CARTESIAN_POINT('',(3.9,0.62,0.));
#11914=CARTESIAN_POINT('',(3.9,0.62,0.32));
#11915=CARTESIAN_POINT('',(3.9,0.62,0.16));
#11916=CARTESIAN_POINT('',(4.1,0.62,0.));
#11917=CARTESIAN_POINT('',(2.98987299740311,0.62,0.));
#11918=CARTESIAN_POINT('',(4.1,0.62,0.32));
#11919=CARTESIAN_POINT('',(4.1,0.62,0.16));
#11920=CARTESIAN_POINT('',(11.2,0.62,0.32));
#11921=CARTESIAN_POINT('Origin',(5.55,0.,0.32));
#11922=CARTESIAN_POINT('',(1.6,-4.89858719658941E-17,0.32));
#11923=CARTESIAN_POINT('Origin',(2.,0.,0.32));
#11924=CARTESIAN_POINT('Origin',(5.55,0.,0.32));
#11925=CARTESIAN_POINT('',(9.6,-4.89858719658942E-17,0.32));
#11926=CARTESIAN_POINT('Origin',(10.,0.,0.32));
#11927=CARTESIAN_POINT('Origin',(5.55,0.,0.32));
#11928=CARTESIAN_POINT('',(0.217044958570157,-0.7,0.32));
#11929=CARTESIAN_POINT('',(0.0167704893705731,-0.7,0.32));
#11930=CARTESIAN_POINT('Origin',(5.55,0.,0.32));
#11931=CARTESIAN_POINT('',(0.9,0.724814814814815,0.32));
#11932=CARTESIAN_POINT('',(1.1,-0.724814814814815,0.32));
#11933=CARTESIAN_POINT('Origin',(5.55,0.,0.32));
#11934=CARTESIAN_POINT('',(3.9,0.883148148148148,0.32));
#11935=CARTESIAN_POINT('',(4.1,-0.883148148148148,0.32));
#11936=CARTESIAN_POINT('Origin',(5.55,0.,0.32));
#11937=CARTESIAN_POINT('',(7.9,0.62,0.32));
#11938=CARTESIAN_POINT('',(7.9,0.886851851851852,0.32));
#11939=CARTESIAN_POINT('',(8.1,0.62,0.32));
#11940=CARTESIAN_POINT('',(11.2,0.62,0.32));
#11941=CARTESIAN_POINT('',(8.1,-0.886851851851852,0.32));
#11942=CARTESIAN_POINT('Origin',(-0.0999999999999996,0.62,0.32));
#11943=CARTESIAN_POINT('',(7.9,0.62,0.));
#11944=CARTESIAN_POINT('',(7.9,0.62,0.16));
#11945=CARTESIAN_POINT('',(8.1,0.62,0.));
#11946=CARTESIAN_POINT('',(2.98987299740311,0.62,0.));
#11947=CARTESIAN_POINT('',(8.1,0.62,0.16));
#11948=CARTESIAN_POINT('Origin',(11.2,1.53779953703704,0.));
#11949=CARTESIAN_POINT('',(11.2,1.47592264243751,0.));
#11950=CARTESIAN_POINT('',(11.2,-1.47592264243751,0.));
#11951=CARTESIAN_POINT('',(11.2,1.53779953703704,0.));
#11952=CARTESIAN_POINT('',(11.2,-1.44160695250311,0.605635447211793));
#11953=CARTESIAN_POINT('Ctrl Pts',(11.2,-1.44160695250311,0.605635447211793));
#11954=CARTESIAN_POINT('Ctrl Pts',(11.2,-1.44733381480461,0.504614841520655));
#11955=CARTESIAN_POINT('Ctrl Pts',(11.2,-1.45305922122436,0.403593539811385));
#11956=CARTESIAN_POINT('Ctrl Pts',(11.2,-1.46449774781658,0.201715464978033));
#11957=CARTESIAN_POINT('Ctrl Pts',(11.2,-1.47021094199039,0.100857470386242));
#11958=CARTESIAN_POINT('Ctrl Pts',(11.2,-1.47592264243751,0.));
#11959=CARTESIAN_POINT('',(11.2,-1.3413305091784,0.7));
#11960=CARTESIAN_POINT('Ctrl Pts',(11.2,-1.34133050917871,0.7));
#11961=CARTESIAN_POINT('Ctrl Pts',(11.2,-1.34927184579059,0.7));
#11962=CARTESIAN_POINT('Ctrl Pts',(11.1999981201149,-1.35715077597425,0.699006225306896));
#11963=CARTESIAN_POINT('Ctrl Pts',(11.1999964866412,-1.36482619101963,0.697118463987577));
#11964=CARTESIAN_POINT('Ctrl Pts',(11.1999955714568,-1.36912648693643,0.696060810134936));
#11965=CARTESIAN_POINT('Ctrl Pts',(11.1999947385598,-1.37336294684024,0.694721504600825));
#11966=CARTESIAN_POINT('Ctrl Pts',(11.1999942054834,-1.37750904339755,0.693111246644731));
#11967=CARTESIAN_POINT('Ctrl Pts',(11.1999932489192,-1.38494889279378,0.690221763364053));
#11968=CARTESIAN_POINT('Ctrl Pts',(11.1999934335488,-1.39201911070639,0.686493604183975));
#11969=CARTESIAN_POINT('Ctrl Pts',(11.1999946360439,-1.39857284316731,0.682006025455124));
#11970=CARTESIAN_POINT('Ctrl Pts',(11.1999952980149,-1.40218065925828,0.679535622697003));
#11971=CARTESIAN_POINT('Ctrl Pts',(11.1999962427007,-1.40563167682227,0.676834205328214));
#11972=CARTESIAN_POINT('Ctrl Pts',(11.1999970766466,-1.40889738828709,0.673909521834337));
#11973=CARTESIAN_POINT('Ctrl Pts',(11.1999978839828,-1.41205889660265,0.671078159882768));
#11974=CARTESIAN_POINT('Ctrl Pts',(11.1999985961359,-1.41502771690814,0.668054510912379));
#11975=CARTESIAN_POINT('Ctrl Pts',(11.1999985943254,-1.41778154893794,0.664849526385156));
#11976=CARTESIAN_POINT('Ctrl Pts',(11.1999985909468,-1.42292039881534,0.658868793295219));
#11977=CARTESIAN_POINT('Ctrl Pts',(11.1999963776609,-1.42731355725865,0.652257958652517));
#11978=CARTESIAN_POINT('Ctrl Pts',(11.1999956369,-1.43089859237711,0.645180832176479));
#11979=CARTESIAN_POINT('Ctrl Pts',(11.1999955610412,-1.43126572346771,0.644456088045497));
#11980=CARTESIAN_POINT('Ctrl Pts',(11.1999954968237,-1.43162433912915,0.643726434786758));
#11981=CARTESIAN_POINT('Ctrl Pts',(11.1999954455063,-1.43197434355081,0.642992037678167));
#11982=CARTESIAN_POINT('Ctrl Pts',(11.1999949451572,-1.43538691836834,0.635831599341589));
#11983=CARTESIAN_POINT('Ctrl Pts',(11.1999960935741,-1.43794480573841,0.628305806294037));
#11984=CARTESIAN_POINT('Ctrl Pts',(11.1999977538348,-1.43959303921538,0.620581877990282));
#11985=CARTESIAN_POINT('Ctrl Pts',(11.1999988103007,-1.44064185190664,0.615666946856702));
#11986=CARTESIAN_POINT('Ctrl Pts',(11.1999999935832,-1.44132148083109,0.610671141596651));
#11987=CARTESIAN_POINT('Ctrl Pts',(11.1999999950647,-1.44160695392865,0.605635447210179));
#11988=CARTESIAN_POINT('',(11.2,1.34133050917871,0.7));
#11989=CARTESIAN_POINT('',(11.2,0.768899768518519,0.7));
#11990=CARTESIAN_POINT('',(11.2,1.44160695250311,0.605635447211793));
#11991=CARTESIAN_POINT('Ctrl Pts',(11.1999999950647,1.44160695392865,0.605635447210179));
#11992=CARTESIAN_POINT('Ctrl Pts',(11.1999999927383,1.44115867123275,0.613543073794128));
#11993=CARTESIAN_POINT('Ctrl Pts',(11.199997327584,1.43974095598264,0.62135504174347));
#11994=CARTESIAN_POINT('Ctrl Pts',(11.1999961426836,1.43743894790867,0.628911795513178));
#11995=CARTESIAN_POINT('Ctrl Pts',(11.1999954950047,1.43618064644969,0.633042395401645));
#11996=CARTESIAN_POINT('Ctrl Pts',(11.1999951984378,1.4346571631488,0.63709676955888));
#11997=CARTESIAN_POINT('Ctrl Pts',(11.1999953420225,1.43287614971348,0.641047046155727));
#11998=CARTESIAN_POINT('Ctrl Pts',(11.1999956050472,1.42961361303411,0.648283331988978));
#11999=CARTESIAN_POINT('Ctrl Pts',(11.1999975633633,1.42552584716917,0.655091209244077));
#12000=CARTESIAN_POINT('Ctrl Pts',(11.1999983488166,1.42067941835906,0.661308913390503));
#12001=CARTESIAN_POINT('Ctrl Pts',(11.1999985007599,1.41974189284539,0.662511707551344));
#12002=CARTESIAN_POINT('Ctrl Pts',(11.1999985958742,1.41877583892185,0.663692344451305));
#12003=CARTESIAN_POINT('Ctrl Pts',(11.1999985956185,1.41778154881703,0.664849526385225));
#12004=CARTESIAN_POINT('Ctrl Pts',(11.199998595152,1.41596832836708,0.666959801783445));
#12005=CARTESIAN_POINT('Ctrl Pts',(11.1999982799021,1.41406123008998,0.668992111776222));
#12006=CARTESIAN_POINT('Ctrl Pts',(11.1999978412043,1.41206657472189,0.670943322037058));
#12007=CARTESIAN_POINT('Ctrl Pts',(11.1999965906985,1.40638082038708,0.676505236328724));
#12008=CARTESIAN_POINT('Ctrl Pts',(11.1999945592311,1.40005057587654,0.681348449922958));
#12009=CARTESIAN_POINT('Ctrl Pts',(11.1999938793032,1.39324090595796,0.685420973467861));
#12010=CARTESIAN_POINT('Ctrl Pts',(11.1999934424014,1.38886521116801,0.68803785802621));
#12011=CARTESIAN_POINT('Ctrl Pts',(11.1999934711477,1.38429057260668,0.690335857752236));
#12012=CARTESIAN_POINT('Ctrl Pts',(11.1999939665515,1.37955471147715,0.692291686537622));
#12013=CARTESIAN_POINT('Ctrl Pts',(11.1999947349645,1.37220899016913,0.695325342464331));
#12014=CARTESIAN_POINT('Ctrl Pts',(11.1999966395725,1.36455954597093,0.697503651902993));
#12015=CARTESIAN_POINT('Ctrl Pts',(11.1999981885915,1.35675452105021,0.698758058199902));
#12016=CARTESIAN_POINT('Ctrl Pts',(11.1999991983045,1.35166689148409,0.699575730741489));
#12017=CARTESIAN_POINT('Ctrl Pts',(11.2,1.34651254223162,0.7));
#12018=CARTESIAN_POINT('Ctrl Pts',(11.2,1.34133050917871,0.7));
#12019=CARTESIAN_POINT('Ctrl Pts',(11.2,1.47592264243751,0.));
#12020=CARTESIAN_POINT('Ctrl Pts',(11.2,1.47021025951677,0.100869521536925));
#12021=CARTESIAN_POINT('Ctrl Pts',(11.2,1.4644963825062,0.20173956751342));
#12022=CARTESIAN_POINT('Ctrl Pts',(11.2,1.45305785520703,0.403617642353031));
#12023=CARTESIAN_POINT('Ctrl Pts',(11.2,1.44733313162379,0.50462689268162));
#12024=CARTESIAN_POINT('Ctrl Pts',(11.2,1.44160695250311,0.605635447211793));
#12025=CARTESIAN_POINT('Origin',(8.1,-1.7737037037037,0.));
#12026=CARTESIAN_POINT('',(8.1,1.69866351109718,0.));
#12027=CARTESIAN_POINT('',(8.1,-1.7737037037037,0.));
#12028=CARTESIAN_POINT('',(8.1,1.66641703131627,0.605314487869832));
#12029=CARTESIAN_POINT('Ctrl Pts',(8.1,1.66641703131627,0.605314487869832));
#12030=CARTESIAN_POINT('Ctrl Pts',(8.1,1.67178339996556,0.504592280948055));
#12031=CARTESIAN_POINT('Ctrl Pts',(8.1,1.67714947719849,0.403869246528492));
#12032=CARTESIAN_POINT('Ctrl Pts',(8.1,1.68789827452893,0.202098297941347));
#12033=CARTESIAN_POINT('Ctrl Pts',(8.1,1.69328107955938,0.101048748975501));
#12034=CARTESIAN_POINT('Ctrl Pts',(8.1,1.69866351109718,0.));
#12035=CARTESIAN_POINT('',(8.1,1.56644778183753,0.7));
#12036=CARTESIAN_POINT('Ctrl Pts',(8.0999999986552,1.56644778212326,0.7));
#12037=CARTESIAN_POINT('Ctrl Pts',(8.10000000155239,1.57436337254628,0.699999999341293));
#12038=CARTESIAN_POINT('Ctrl Pts',(8.09999905041684,1.58221543358893,0.699005989267703));
#12039=CARTESIAN_POINT('Ctrl Pts',(8.09999821745812,1.58986365929578,0.697118696434997));
#12040=CARTESIAN_POINT('Ctrl Pts',(8.099997748439,1.59417019217574,0.69605600700222));
#12041=CARTESIAN_POINT('Ctrl Pts',(8.09999731997616,1.59841215407948,0.694709061504878));
#12042=CARTESIAN_POINT('Ctrl Pts',(8.09999704681388,1.60256279759721,0.693088866918468));
#12043=CARTESIAN_POINT('Ctrl Pts',(8.09999655811104,1.60998853482381,0.690190246691698));
#12044=CARTESIAN_POINT('Ctrl Pts',(8.09999665589197,1.61704187682962,0.686451534538094));
#12045=CARTESIAN_POINT('Ctrl Pts',(8.09999726576867,1.62357667434142,0.681954089017224));
#12046=CARTESIAN_POINT('Ctrl Pts',(8.09999760196939,1.62717904774802,0.679474826559159));
#12047=CARTESIAN_POINT('Ctrl Pts',(8.09999808150314,1.6306235748906,0.676764109620253));
#12048=CARTESIAN_POINT('Ctrl Pts',(8.09999850764167,1.63388182210815,0.673830012183301));
#12049=CARTESIAN_POINT('Ctrl Pts',(8.09999892160867,1.637047006066,0.670979719520364));
#12050=CARTESIAN_POINT('Ctrl Pts',(8.09999928906958,1.640017230617,0.667935813742119));
#12051=CARTESIAN_POINT('Ctrl Pts',(8.09999928944056,1.64277007752663,0.664709670235875));
#12052=CARTESIAN_POINT('Ctrl Pts',(8.09999929012967,1.64788359851353,0.658716982277737));
#12053=CARTESIAN_POINT('Ctrl Pts',(8.09999816327153,1.65225000627493,0.652096887528603));
#12054=CARTESIAN_POINT('Ctrl Pts',(8.09999778355904,1.65580927004486,0.645014643130784));
#12055=CARTESIAN_POINT('Ctrl Pts',(8.09999774450894,1.65617530914943,0.644286296325024));
#12056=CARTESIAN_POINT('Ctrl Pts',(8.09999771143612,1.65653277094855,0.643553041785202));
#12057=CARTESIAN_POINT('Ctrl Pts',(8.0999976850083,1.65688156115921,0.642815048027137));
#12058=CARTESIAN_POINT('Ctrl Pts',(8.09999742811004,1.66027206465027,0.635641192980042));
#12059=CARTESIAN_POINT('Ctrl Pts',(8.09999800724182,1.66280786743682,0.628104262855387));
#12060=CARTESIAN_POINT('Ctrl Pts',(8.09999885110511,1.66443535430957,0.620372450280339));
#12061=CARTESIAN_POINT('Ctrl Pts',(8.09999939164969,1.6654778563549,0.615419764910946));
#12062=CARTESIAN_POINT('Ctrl Pts',(8.1,1.66614680274328,0.610386449940169));
#12063=CARTESIAN_POINT('Ctrl Pts',(8.1,1.66641703131627,0.605314487869832));
#12064=CARTESIAN_POINT('',(8.1,-1.56644778183827,0.7));
#12065=CARTESIAN_POINT('',(8.1,-0.886851851851852,0.7));
#12066=CARTESIAN_POINT('',(8.1,-1.66641703131627,0.605314487869832));
#12067=CARTESIAN_POINT('Ctrl Pts',(8.1,-1.66641703131627,0.605314487869832));
#12068=CARTESIAN_POINT('Ctrl Pts',(8.1,-1.66599546653325,0.613226902778437));
#12069=CARTESIAN_POINT('Ctrl Pts',(8.09999864563672,-1.66460605882141,0.621047760783158));
#12070=CARTESIAN_POINT('Ctrl Pts',(8.09999804140045,-1.66233302739118,0.628616817026045));
#12071=CARTESIAN_POINT('Ctrl Pts',(8.09999770486592,-1.66106704316887,0.632832467392296));
#12072=CARTESIAN_POINT('Ctrl Pts',(8.0999975536836,-1.65952595995304,0.636970042829054));
#12073=CARTESIAN_POINT('Ctrl Pts',(8.09999763427866,-1.65771765414013,0.640999885518982));
#12074=CARTESIAN_POINT('Ctrl Pts',(8.09999777898787,-1.65447082344915,0.64823550729937));
#12075=CARTESIAN_POINT('Ctrl Pts',(8.09999878245444,-1.65040085231772,0.655045563401426));
#12076=CARTESIAN_POINT('Ctrl Pts',(8.09999917121848,-1.64557198994432,0.661267087195486));
#12077=CARTESIAN_POINT('Ctrl Pts',(8.09999924425118,-1.6446648462537,0.662435854416292));
#12078=CARTESIAN_POINT('Ctrl Pts',(8.09999928944999,-1.64373079085321,0.663583781603691));
#12079=CARTESIAN_POINT('Ctrl Pts',(8.09999928890117,-1.64277007755202,0.664709670235858));
#12080=CARTESIAN_POINT('Ctrl Pts',(8.09999928782175,-1.64088054556816,0.666924069243459));
#12081=CARTESIAN_POINT('Ctrl Pts',(8.09999911129818,-1.63888792496677,0.66905326411728));
#12082=CARTESIAN_POINT('Ctrl Pts',(8.09999887085824,-1.63679941630975,0.671093569621172));
#12083=CARTESIAN_POINT('Ctrl Pts',(8.09999821641022,-1.6311147520694,0.676647030794692));
#12084=CARTESIAN_POINT('Ctrl Pts',(8.0999972000003,-1.62478663867955,0.681482189379454));
#12085=CARTESIAN_POINT('Ctrl Pts',(8.09999686812141,-1.6179789612855,0.685544965666037));
#12086=CARTESIAN_POINT('Ctrl Pts',(8.09999665686968,-1.61364565292072,0.68813105508359));
#12087=CARTESIAN_POINT('Ctrl Pts',(8.09999667786582,-1.6091170759025,0.690403516124292));
#12088=CARTESIAN_POINT('Ctrl Pts',(8.0999969341683,-1.60442977212996,0.692339085768374));
#12089=CARTESIAN_POINT('Ctrl Pts',(8.09999733452329,-1.59710801128849,0.695362524980696));
#12090=CARTESIAN_POINT('Ctrl Pts',(8.09999831212369,-1.58948382509795,0.697531565976904));
#12091=CARTESIAN_POINT('Ctrl Pts',(8.09999909563861,-1.58170429192971,0.698776637084609));
#12092=CARTESIAN_POINT('Ctrl Pts',(8.09999960249138,-1.57667174192468,0.69958206878261));
#12093=CARTESIAN_POINT('Ctrl Pts',(8.1000000005313,-1.5715735875011,0.699999999573449));
#12094=CARTESIAN_POINT('Ctrl Pts',(8.0999999986552,-1.56644778212326,0.7));
#12095=CARTESIAN_POINT('',(8.1,-1.69866351109718,0.));
#12096=CARTESIAN_POINT('Ctrl Pts',(8.1,-1.69866351109718,0.));
#12097=CARTESIAN_POINT('Ctrl Pts',(8.1,-1.69328105674055,0.101049177371948));
#12098=CARTESIAN_POINT('Ctrl Pts',(8.1,-1.68789822886868,0.202099155105557));
#12099=CARTESIAN_POINT('Ctrl Pts',(8.1,-1.67714943151225,0.403870104074094));
#12100=CARTESIAN_POINT('Ctrl Pts',(8.1,-1.67178337712185,0.50459270970527));
#12101=CARTESIAN_POINT('Ctrl Pts',(8.1,-1.66641703131627,0.605314487869832));
#12102=CARTESIAN_POINT('',(8.1,-1.7737037037037,0.));
#12103=CARTESIAN_POINT('Origin',(4.1,-1.7662962962963,0.));
#12104=CARTESIAN_POINT('',(4.1,1.70113889814581,0.));
#12105=CARTESIAN_POINT('',(4.1,-1.7662962962963,0.));
#12106=CARTESIAN_POINT('',(4.1,1.66887738702937,0.605315322680072));
#12107=CARTESIAN_POINT('Ctrl Pts',(4.1,1.66887738702937,0.605315322680072));
#12108=CARTESIAN_POINT('Ctrl Pts',(4.1,1.67424235111642,0.50466767694528));
#12109=CARTESIAN_POINT('Ctrl Pts',(4.1,1.67960699363804,0.404019058341251));
#12110=CARTESIAN_POINT('Ctrl Pts',(4.1,1.69036079691899,0.202247931921761));
#12111=CARTESIAN_POINT('Ctrl Pts',(4.1,1.6957500571643,0.101123491803998));
#12112=CARTESIAN_POINT('Ctrl Pts',(4.1,1.70113889814581,0.));
#12113=CARTESIAN_POINT('',(4.1,1.56887583540973,0.7));
#12114=CARTESIAN_POINT('Ctrl Pts',(4.1,1.56887583540973,0.7));
#12115=CARTESIAN_POINT('Ctrl Pts',(4.1,1.57679416129392,0.7));
#12116=CARTESIAN_POINT('Ctrl Pts',(4.10000107724674,1.58464912207822,0.699006028000541));
#12117=CARTESIAN_POINT('Ctrl Pts',(4.10000201939527,1.59230028572239,0.697118705459362));
#12118=CARTESIAN_POINT('Ctrl Pts',(4.10000255022779,1.59661116283941,0.696055335763773));
#12119=CARTESIAN_POINT('Ctrl Pts',(4.10000303435977,1.60085740028891,0.694707333985525));
#12120=CARTESIAN_POINT('Ctrl Pts',(4.10000334030352,1.60501217339351,0.693085708041268));
#12121=CARTESIAN_POINT('Ctrl Pts',(4.10000388718746,1.61243895913315,0.690187001388783));
#12122=CARTESIAN_POINT('Ctrl Pts',(4.10000376557609,1.61949349263125,0.686448444730844));
#12123=CARTESIAN_POINT('Ctrl Pts',(4.10000306534783,1.6260295229635,0.681951159450519));
#12124=CARTESIAN_POINT('Ctrl Pts',(4.10000267892397,1.62963645835533,0.679469313954069));
#12125=CARTESIAN_POINT('Ctrl Pts',(4.10000213012555,1.63308521926452,0.676755517937216));
#12126=CARTESIAN_POINT('Ctrl Pts',(4.1000016436875,1.63634725251217,0.673817835781739));
#12127=CARTESIAN_POINT('Ctrl Pts',(4.10000117237165,1.63950787692018,0.67097147916344));
#12128=CARTESIAN_POINT('Ctrl Pts',(4.10000075597222,1.64247408874941,0.667932078875657));
#12129=CARTESIAN_POINT('Ctrl Pts',(4.10000075698646,1.64522354659423,0.664710927554201));
#12130=CARTESIAN_POINT('Ctrl Pts',(4.1000007588733,1.65033845220459,0.658718515269377));
#12131=CARTESIAN_POINT('Ctrl Pts',(4.10000204656096,1.65470614797426,0.652098486008568));
#12132=CARTESIAN_POINT('Ctrl Pts',(4.10000248678323,1.65826650381873,0.645016049251367));
#12133=CARTESIAN_POINT('Ctrl Pts',(4.10000253228732,1.65863452415637,0.644283964909082));
#12134=CARTESIAN_POINT('Ctrl Pts',(4.10000257095464,1.65899387729575,0.643546919913709));
#12135=CARTESIAN_POINT('Ctrl Pts',(4.10000260201855,1.65934446736461,0.642805085364403));
#12136=CARTESIAN_POINT('Ctrl Pts',(4.10000290242009,1.66273482600052,0.635631222228741));
#12137=CARTESIAN_POINT('Ctrl Pts',(4.10000225562543,1.66527033938482,0.628094305374488));
#12138=CARTESIAN_POINT('Ctrl Pts',(4.10000130084992,1.66689736875237,0.62036252267401));
#12139=CARTESIAN_POINT('Ctrl Pts',(4.10000068968835,1.66793884687677,0.615413329558163));
#12140=CARTESIAN_POINT('Ctrl Pts',(4.09999999901039,1.66860722297681,0.610383627857512));
#12141=CARTESIAN_POINT('Ctrl Pts',(4.09999999630223,1.66887738567036,0.60531532268817));
#12142=CARTESIAN_POINT('',(4.1,-1.56887583540947,0.7));
#12143=CARTESIAN_POINT('',(4.1,-0.883148148148148,0.7));
#12144=CARTESIAN_POINT('',(4.1,-1.66887738702937,0.605315322680072));
#12145=CARTESIAN_POINT('Ctrl Pts',(4.09999999630223,-1.66887738567036,0.60531532268817));
#12146=CARTESIAN_POINT('Ctrl Pts',(4.10000000053001,-1.66845562780346,0.613227583070809));
#12147=CARTESIAN_POINT('Ctrl Pts',(4.10000153668442,-1.66706589531621,0.621048261667561));
#12148=CARTESIAN_POINT('Ctrl Pts',(4.10000221487211,-1.66479240287642,0.628617079688242));
#12149=CARTESIAN_POINT('Ctrl Pts',(4.10000259231836,-1.6635270876889,0.632829515245766));
#12150=CARTESIAN_POINT('Ctrl Pts',(4.10000275805793,-1.66198703315979,0.636963972243471));
#12151=CARTESIAN_POINT('Ctrl Pts',(4.10000266178038,-1.66018010017296,0.640990858692597));
#12152=CARTESIAN_POINT('Ctrl Pts',(4.10000248876893,-1.65693302887506,0.648227201990446));
#12153=CARTESIAN_POINT('Ctrl Pts',(4.10000134097948,-1.65286254930452,0.655037795911226));
#12154=CARTESIAN_POINT('Ctrl Pts',(4.100000893742,-1.6480330317196,0.661259713776781));
#12155=CARTESIAN_POINT('Ctrl Pts',(4.10000080951506,-1.647123502594,0.662431469633614));
#12156=CARTESIAN_POINT('Ctrl Pts',(4.10000075717637,-1.6461869221106,0.663582276554164));
#12157=CARTESIAN_POINT('Ctrl Pts',(4.10000075728519,-1.64522354661022,0.66471092755419));
#12158=CARTESIAN_POINT('Ctrl Pts',(4.10000075749815,-1.64333815989002,0.666919768869269));
#12159=CARTESIAN_POINT('Ctrl Pts',(4.1000009568795,-1.64135017761634,0.669043797975229));
#12160=CARTESIAN_POINT('Ctrl Pts',(4.10000122972053,-1.63926675509047,0.671079366787198));
#12161=CARTESIAN_POINT('Ctrl Pts',(4.10000197419082,-1.6335819569127,0.676633591976433));
#12162=CARTESIAN_POINT('Ctrl Pts',(4.10000313643093,-1.62725355063421,0.681469444454218));
#12163=CARTESIAN_POINT('Ctrl Pts',(4.1000035230587,-1.62044557755217,0.685533082105531));
#12164=CARTESIAN_POINT('Ctrl Pts',(4.10000376939409,-1.61610795658125,0.688122181633714));
#12165=CARTESIAN_POINT('Ctrl Pts',(4.10000375220654,-1.61157469281532,0.690397125746379));
#12166=CARTESIAN_POINT('Ctrl Pts',(4.10000346632868,-1.60688245467732,0.692334655286926));
#12167=CARTESIAN_POINT('Ctrl Pts',(4.10000302008581,-1.59955807566073,0.695359054367588));
#12168=CARTESIAN_POINT('Ctrl Pts',(4.1000019139068,-1.59193114173487,0.69752894708864));
#12169=CARTESIAN_POINT('Ctrl Pts',(4.10000102635309,-1.58414888227482,0.698774888159427));
#12170=CARTESIAN_POINT('Ctrl Pts',(4.10000045177616,-1.57911086966871,0.699581474839467));
#12171=CARTESIAN_POINT('Ctrl Pts',(4.1,-1.57400716417114,0.7));
#12172=CARTESIAN_POINT('Ctrl Pts',(4.1,-1.56887583540973,0.7));
#12173=CARTESIAN_POINT('',(4.1,-1.70113889814582,0.));
#12174=CARTESIAN_POINT('Ctrl Pts',(4.1,-1.70113889814582,0.));
#12175=CARTESIAN_POINT('Ctrl Pts',(4.1,-1.69575004793467,0.101123665001254));
#12176=CARTESIAN_POINT('Ctrl Pts',(4.1,-1.69036077845691,0.202248278345555));
#12177=CARTESIAN_POINT('Ctrl Pts',(4.1,-1.67960697517202,0.404019404791024));
#12178=CARTESIAN_POINT('Ctrl Pts',(4.1,-1.67424234188296,0.504667850166609));
#12179=CARTESIAN_POINT('Ctrl Pts',(4.1,-1.66887738702937,0.605315322680072));
#12180=CARTESIAN_POINT('',(4.1,-1.7662962962963,0.));
#12181=CARTESIAN_POINT('Origin',(1.1,-1.44962962962963,0.));
#12182=CARTESIAN_POINT('',(1.1,1.39262953588351,0.));
#12183=CARTESIAN_POINT('',(1.1,-1.44962962962963,0.));
#12184=CARTESIAN_POINT('',(1.10000000000005,1.35674377243284,0.605845626926786));
#12185=CARTESIAN_POINT('Ctrl Pts',(1.10000000000005,1.35674377243284,0.605845626926786));
#12186=CARTESIAN_POINT('Ctrl Pts',(1.10000000000005,1.36273568520883,0.504787121979256));
#12187=CARTESIAN_POINT('Ctrl Pts',(1.1,1.36872466312622,0.403727404115485));
#12188=CARTESIAN_POINT('Ctrl Pts',(1.1,1.38068651056748,0.201779555185378));
#12189=CARTESIAN_POINT('Ctrl Pts',(1.1,1.38665951284069,0.10088935150083));
#12190=CARTESIAN_POINT('Ctrl Pts',(1.1,1.39262953588351,0.));
#12191=CARTESIAN_POINT('',(1.1,1.25565664448622,0.7));
#12192=CARTESIAN_POINT('Ctrl Pts',(1.1,1.25565664448621,0.7));
#12193=CARTESIAN_POINT('Ctrl Pts',(1.1,1.26365753466764,0.700000000000001));
#12194=CARTESIAN_POINT('Ctrl Pts',(1.10000312127109,1.27160078819195,0.699008097631352));
#12195=CARTESIAN_POINT('Ctrl Pts',(1.10000579554281,1.27934333527045,0.697120485426804));
#12196=CARTESIAN_POINT('Ctrl Pts',(1.10000709386889,1.28310224676699,0.696204072889075));
#12197=CARTESIAN_POINT('Ctrl Pts',(1.10000828779753,1.28681383019745,0.695075712339665));
#12198=CARTESIAN_POINT('Ctrl Pts',(1.10000913303706,1.29046059826345,0.693742188764313));
#12199=CARTESIAN_POINT('Ctrl Pts',(1.10001087659788,1.29798315455626,0.69099139518989));
#12200=CARTESIAN_POINT('Ctrl Pts',(1.10001086910546,1.30515375246939,0.687398976275641));
#12201=CARTESIAN_POINT('Ctrl Pts',(1.10000899624477,1.31182501206943,0.683041610144935));
#12202=CARTESIAN_POINT('Ctrl Pts',(1.10000779407289,1.31610723164143,0.680244657298552));
#12203=CARTESIAN_POINT('Ctrl Pts',(1.10000585478529,1.32018349952736,0.677131483611404));
#12204=CARTESIAN_POINT('Ctrl Pts',(1.10000422180804,1.32400796947387,0.673713330684339));
#12205=CARTESIAN_POINT('Ctrl Pts',(1.10000291018178,1.3270798280974,0.670967830603965));
#12206=CARTESIAN_POINT('Ctrl Pts',(1.10000180047651,1.32997084712789,0.668041731908725));
#12207=CARTESIAN_POINT('Ctrl Pts',(1.10000182449184,1.33266034096938,0.664944387470286));
#12208=CARTESIAN_POINT('Ctrl Pts',(1.10000187074845,1.33784065079383,0.65897850512594));
#12209=CARTESIAN_POINT('Ctrl Pts',(1.10000564109429,1.34227630326151,0.652378581761819));
#12210=CARTESIAN_POINT('Ctrl Pts',(1.10000696187003,1.34590032739451,0.645305437365917));
#12211=CARTESIAN_POINT('Ctrl Pts',(1.100007110355,1.34630774940504,0.644510256482779));
#12212=CARTESIAN_POINT('Ctrl Pts',(1.10000723579819,1.34670486410349,0.643709073603569));
#12213=CARTESIAN_POINT('Ctrl Pts',(1.10000733566964,1.34709153749004,0.642902104572485));
#12214=CARTESIAN_POINT('Ctrl Pts',(1.10000822022419,1.35051627708745,0.63575483535061));
#12215=CARTESIAN_POINT('Ctrl Pts',(1.10000635568239,1.35308446649167,0.628241602461225));
#12216=CARTESIAN_POINT('Ctrl Pts',(1.10000361780323,1.35473867947858,0.620527690691125));
#12217=CARTESIAN_POINT('Ctrl Pts',(1.1000019043033,1.35577396762308,0.615699943921843));
#12218=CARTESIAN_POINT('Ctrl Pts',(1.09999998677418,1.35645041192828,0.610792997969602));
#12219=CARTESIAN_POINT('Ctrl Pts',(1.09999997754868,1.35674374570294,0.605845627052288));
#12220=CARTESIAN_POINT('',(1.1,-1.25565664448622,0.7));
#12221=CARTESIAN_POINT('',(1.1,-0.724814814814815,0.7));
#12222=CARTESIAN_POINT('',(1.10000000000005,-1.35674377243284,0.605845626926786));
#12223=CARTESIAN_POINT('Ctrl Pts',(1.09999997754868,-1.35674374570294,0.605845627052288));
#12224=CARTESIAN_POINT('Ctrl Pts',(1.09999999227748,-1.35627542940044,0.613744255356351));
#12225=CARTESIAN_POINT('Ctrl Pts',(1.1000044245081,-1.35483313756702,0.621542702113576));
#12226=CARTESIAN_POINT('Ctrl Pts',(1.10000632213307,-1.3525036790266,0.629082464357584));
#12227=CARTESIAN_POINT('Ctrl Pts',(1.1000073336739,-1.3512619466217,0.633101581650771));
#12228=CARTESIAN_POINT('Ctrl Pts',(1.10000777634458,-1.34976719347553,0.637047225321331));
#12229=CARTESIAN_POINT('Ctrl Pts',(1.10000752568741,-1.34802684471036,0.640893844816285));
#12230=CARTESIAN_POINT('Ctrl Pts',(1.10000705344834,-1.3447480208661,0.648140890909733));
#12231=CARTESIAN_POINT('Ctrl Pts',(1.10000374385205,-1.34063788586045,0.654954534019122));
#12232=CARTESIAN_POINT('Ctrl Pts',(1.10000230512149,-1.33576793982513,0.661175616324976));
#12233=CARTESIAN_POINT('Ctrl Pts',(1.10000200863552,-1.33476436716076,0.662457623989879));
#12234=CARTESIAN_POINT('Ctrl Pts',(1.10000181701501,-1.33372836971272,0.663714393476354));
#12235=CARTESIAN_POINT('Ctrl Pts',(1.10000180919237,-1.33266033853372,0.664944387472089));
#12236=CARTESIAN_POINT('Ctrl Pts',(1.10000179685332,-1.33097567746633,0.666884520904953));
#12237=CARTESIAN_POINT('Ctrl Pts',(1.10000223926429,-1.32921133126375,0.668758058859172));
#12238=CARTESIAN_POINT('Ctrl Pts',(1.10000288715521,-1.32737234926393,0.670562692084704));
#12239=CARTESIAN_POINT('Ctrl Pts',(1.10000489069569,-1.32168547392559,0.676143347135183));
#12240=CARTESIAN_POINT('Ctrl Pts',(1.10000845923633,-1.31535192007569,0.681005160308095));
#12241=CARTESIAN_POINT('Ctrl Pts',(1.1000097672184,-1.30853956043085,0.685101187995272));
#12242=CARTESIAN_POINT('Ctrl Pts',(1.10001062829021,-1.30405484229164,0.687797688271992));
#12243=CARTESIAN_POINT('Ctrl Pts',(1.10001067755751,-1.29936155475819,0.690161668140197));
#12244=CARTESIAN_POINT('Ctrl Pts',(1.10000992106221,-1.29450057597768,0.692169783635984));
#12245=CARTESIAN_POINT('Ctrl Pts',(1.10000876843985,-1.28709422081189,0.695229417764685));
#12246=CARTESIAN_POINT('Ctrl Pts',(1.100005676647,-1.27938091857402,0.69743146309387));
#12247=CARTESIAN_POINT('Ctrl Pts',(1.10000309801581,-1.2715114871423,0.698709794160748));
#12248=CARTESIAN_POINT('Ctrl Pts',(1.10000138449209,-1.26628217885177,0.699559256705032));
#12249=CARTESIAN_POINT('Ctrl Pts',(1.1,-1.26098326598685,0.700000000000001));
#12250=CARTESIAN_POINT('Ctrl Pts',(1.1,-1.25565664448621,0.7));
#12251=CARTESIAN_POINT('',(1.1,-1.39262953588351,0.));
#12252=CARTESIAN_POINT('Ctrl Pts',(1.1,-1.39262953588351,0.));
#12253=CARTESIAN_POINT('Ctrl Pts',(1.1,-1.38665944902278,0.100890429980357));
#12254=CARTESIAN_POINT('Ctrl Pts',(1.1,-1.38068638286488,0.201781712214768));
#12255=CARTESIAN_POINT('Ctrl Pts',(1.1,-1.36872453529477,0.403729561179669));
#12256=CARTESIAN_POINT('Ctrl Pts',(1.10000000000005,-1.3627356212621,0.504788200493074));
#12257=CARTESIAN_POINT('Ctrl Pts',(1.10000000000005,-1.35674377243284,0.605845626926786));
#12258=CARTESIAN_POINT('',(1.1,-1.44962962962963,0.));
#12259=CARTESIAN_POINT('Origin',(0.199725906950915,-1.4,-0.0104671912485888));
#12260=CARTESIAN_POINT('',(0.200274469199584,1.15262458915154,1.38777878078145E-17));
#12261=CARTESIAN_POINT('',(0.200274469199585,-0.7,0.));
#12262=CARTESIAN_POINT('',(0.231993417893744,1.12115139781563,0.605233595624295));
#12263=CARTESIAN_POINT('Ctrl Pts',(0.200274469199584,1.15262458915154,-5.50774703622636E-17));
#12264=CARTESIAN_POINT('Ctrl Pts',(0.210847451072758,1.1421331482829,0.201744512318911));
#12265=CARTESIAN_POINT('Ctrl Pts',(0.221420433966108,1.13164208276446,0.403489044103923));
#12266=CARTESIAN_POINT('Ctrl Pts',(0.231993417893744,1.12115139781563,0.605233595624295));
#12267=CARTESIAN_POINT('',(0.231993417893744,-1.12115139781563,0.605233595624295));
#12268=CARTESIAN_POINT('',(0.231993417893744,-0.7,0.605233595624295));
#12269=CARTESIAN_POINT('',(0.200274469199584,-1.15262458915154,1.38777878078145E-17));
#12270=CARTESIAN_POINT('Ctrl Pts',(0.231993417893744,-1.12115139781563,
0.605233595624295));
#12271=CARTESIAN_POINT('Ctrl Pts',(0.221420433966108,-1.13164208276446,
0.403489044103923));
#12272=CARTESIAN_POINT('Ctrl Pts',(0.210847451072758,-1.1421331482829,0.201744512318911));
#12273=CARTESIAN_POINT('Ctrl Pts',(0.200274469199584,-1.15262458915154,
-6.67868538251071E-17));
#12274=CARTESIAN_POINT('',(0.200274469199585,-0.7,0.));
#12275=CARTESIAN_POINT('Origin',(6.07974599480623,0.,0.));
#12276=CARTESIAN_POINT('Ctrl Pts',(8.1,-1.69866351109718,4.37041895728907E-16));
#12277=CARTESIAN_POINT('Ctrl Pts',(8.9524267631348,-1.65897367198627,1.20944032620455E-7));
#12278=CARTESIAN_POINT('Ctrl Pts',(9.80407798130771,-1.59837060538327,2.76830114922109E-8));
#12279=CARTESIAN_POINT('Ctrl Pts',(10.6537697771985,-1.52488560579501,1.03413542584124E-8));
#12280=CARTESIAN_POINT('Ctrl Pts',(10.8359404901627,-1.50913069933138,6.62336842220622E-9));
#12281=CARTESIAN_POINT('Ctrl Pts',(11.0180211259896,-1.49278349820154,3.93228299510406E-9));
#12282=CARTESIAN_POINT('Ctrl Pts',(11.2000000002909,-1.47592264092474,-3.0227174540096E-11));
#12283=CARTESIAN_POINT('Ctrl Pts',(11.2000000002909,1.47592264092474,-3.02272213335841E-11));
#12284=CARTESIAN_POINT('Ctrl Pts',(10.4240589919717,1.54781576943643,1.68591524001238E-8));
#12285=CARTESIAN_POINT('Ctrl Pts',(9.64626799696257,1.61037563220813,6.17878738288937E-8));
#12286=CARTESIAN_POINT('Ctrl Pts',(8.86753211358286,1.65747704847969,5.27022751808308E-8));
#12287=CARTESIAN_POINT('Ctrl Pts',(8.61177933690776,1.67294611604661,4.97183789310355E-8));
#12288=CARTESIAN_POINT('Ctrl Pts',(8.35592462822135,1.68674740550612,3.63007687033005E-8));
#12289=CARTESIAN_POINT('Ctrl Pts',(8.1,1.69866351109718,3.71000138306103E-16));
#12290=CARTESIAN_POINT('',(7.9,1.70758761671949,0.));
#12291=CARTESIAN_POINT('',(7.9,1.7737037037037,0.));
#12292=CARTESIAN_POINT('Ctrl Pts',(7.90000000036908,1.70758761645525,-3.06814577203155E-11));
#12293=CARTESIAN_POINT('Ctrl Pts',(7.26247716501442,1.73478515342832,3.65175246633048E-8));
#12294=CARTESIAN_POINT('Ctrl Pts',(6.624575449312,1.74993328406844,-3.04558542439636E-7));
#12295=CARTESIAN_POINT('Ctrl Pts',(5.98677261990733,1.74972113442148,-3.1918790057331E-7));
#12296=CARTESIAN_POINT('Ctrl Pts',(5.35540610719671,1.74951112565922,-3.33669628155763E-7));
#12297=CARTESIAN_POINT('Ctrl Pts',(4.72663057529054,1.73425216511322,1.21151810208783E-7));
#12298=CARTESIAN_POINT('Ctrl Pts',(4.10000000045307,1.7011388979176,-4.27317258673188E-11));
#12299=CARTESIAN_POINT('',(3.9,1.68995649764597,0.));
#12300=CARTESIAN_POINT('',(3.9,1.7662962962963,0.));
#12301=CARTESIAN_POINT('Ctrl Pts',(3.9,1.68995649764597,-1.6113354923472E-17));
#12302=CARTESIAN_POINT('Ctrl Pts',(2.96252047830716,1.63464572816558,-1.61179993858831E-17));
#12303=CARTESIAN_POINT('Ctrl Pts',(2.02971500398675,1.53866944530133,-1.61823222708931E-17));
#12304=CARTESIAN_POINT('Ctrl Pts',(1.1,1.39262953588351,-1.60717230190728E-17));
#12305=CARTESIAN_POINT('',(0.9,1.3604297237941,0.));
#12306=CARTESIAN_POINT('',(0.9,1.44962962962963,0.));
#12307=CARTESIAN_POINT('',(0.28146619846596,1.25073018526678,0.));
#12308=CARTESIAN_POINT('Ctrl Pts',(0.899999999999963,1.36042972379409,2.53412200078296E-14));
#12309=CARTESIAN_POINT('Ctrl Pts',(0.693681964344164,1.32640030945436,-1.68820282978727E-7));
#12310=CARTESIAN_POINT('Ctrl Pts',(0.487510176034459,1.28986876146525,1.95094241611213E-11));
#12311=CARTESIAN_POINT('Ctrl Pts',(0.281466198465954,1.25073018526678,9.09211941846344E-16));
#12312=CARTESIAN_POINT('Ctrl Pts',(0.28146619846596,1.25073018526678,4.90059381963448E-17));
#12313=CARTESIAN_POINT('Ctrl Pts',(0.273672142824666,1.24924968434803,-1.60851827685828E-11));
#12314=CARTESIAN_POINT('Ctrl Pts',(0.266112037439191,1.2468180315926,-2.29735811958388E-6));
#12315=CARTESIAN_POINT('Ctrl Pts',(0.258922416881026,1.24354471831116,-3.39045428380668E-6));
#12316=CARTESIAN_POINT('Ctrl Pts',(0.254316658841251,1.24144779416325,-4.09070493067818E-6));
#12317=CARTESIAN_POINT('Ctrl Pts',(0.249862973385875,1.23900427835211,-4.3601744978078E-6));
#12318=CARTESIAN_POINT('Ctrl Pts',(0.245601965247185,1.23623285256398,-4.0505643599354E-6));
#12319=CARTESIAN_POINT('Ctrl Pts',(0.238945660500109,1.23190348870705,-3.5669089987193E-6));
#12320=CARTESIAN_POINT('Ctrl Pts',(0.232836306411817,1.22682685988243,-1.47564048465526E-6));
#12321=CARTESIAN_POINT('Ctrl Pts',(0.227416445112993,1.2210931256102,-3.43092614100725E-7));
#12322=CARTESIAN_POINT('Ctrl Pts',(0.225957664245637,1.21954986437275,-3.82620891408318E-8));
#12323=CARTESIAN_POINT('Ctrl Pts',(0.224549002474426,1.21795876469157,1.76022586487844E-7));
#12324=CARTESIAN_POINT('Ctrl Pts',(0.223193686986583,1.21632111005909,2.01577349231486E-7));
#12325=CARTESIAN_POINT('Ctrl Pts',(0.221344954485829,1.21408724984631,2.36435595047204E-7));
#12326=CARTESIAN_POINT('Ctrl Pts',(0.219595448227346,1.21176677459781,-7.7718209010198E-8));
#12327=CARTESIAN_POINT('Ctrl Pts',(0.217948412504407,1.20936721934621,-5.08402878561E-7));
#12328=CARTESIAN_POINT('Ctrl Pts',(0.213467776427723,1.20283941082417,-1.68004793834142E-6));
#12329=CARTESIAN_POINT('Ctrl Pts',(0.20978887558685,1.19579640990262,-3.43350901357988E-6));
#12330=CARTESIAN_POINT('Ctrl Pts',(0.206958221875648,1.18840352636746,-3.67425174897535E-6));
#12331=CARTESIAN_POINT('Ctrl Pts',(0.206193447398199,1.18640614723908,-3.7392946395744E-6));
#12332=CARTESIAN_POINT('Ctrl Pts',(0.205490847532167,1.18438308363371,-3.7149036306613E-6));
#12333=CARTESIAN_POINT('Ctrl Pts',(0.204851940804359,1.18233735619935,-3.6037364623937E-6));
#12334=CARTESIAN_POINT('Ctrl Pts',(0.202492508448082,1.17478264548698,-3.19320484275276E-6));
#12335=CARTESIAN_POINT('Ctrl Pts',(0.201019195184615,1.16698811697394,-1.36638523817118E-6));
#12336=CARTESIAN_POINT('Ctrl Pts',(0.200491965466086,1.15911075533121,-4.28455138775697E-7));
#12337=CARTESIAN_POINT('Ctrl Pts',(0.200347608840846,1.15695391685535,-1.71647870329038E-7));
#12338=CARTESIAN_POINT('Ctrl Pts',(0.200274469313241,1.15479080601565,-7.49035961899928E-12));
#12339=CARTESIAN_POINT('Ctrl Pts',(0.200274469199584,1.15262458915154,9.10729824887824E-18));
#12340=CARTESIAN_POINT('',(2.01407162049393E-18,1.15316892111334,2.77409355997279E-17));
#12341=CARTESIAN_POINT('',(0.,-1.4,0.));
#12342=CARTESIAN_POINT('',(0.243580684154574,1.44748675362873,2.77555756156289E-17));
#12343=CARTESIAN_POINT('Ctrl Pts',(0.243580684154575,1.44748675362873,-1.56125112837913E-16));
#12344=CARTESIAN_POINT('Ctrl Pts',(0.226022619058538,1.44415189332774,-6.74769223000006E-12));
#12345=CARTESIAN_POINT('Ctrl Pts',(0.208837776424359,1.43922483814223,-1.83343972289099E-6));
#12346=CARTESIAN_POINT('Ctrl Pts',(0.192216855517481,1.43283671850359,-2.37047811876899E-6));
#12347=CARTESIAN_POINT('Ctrl Pts',(0.175448307189507,1.42639185943196,-2.91228650265529E-6));
#12348=CARTESIAN_POINT('Ctrl Pts',(0.15925228528901,1.41845922211561,-2.09168970691363E-6));
#12349=CARTESIAN_POINT('Ctrl Pts',(0.143842215871583,1.4091253227419,-1.20497646612983E-7));
#12350=CARTESIAN_POINT('Ctrl Pts',(0.141154971457358,1.40749765525544,2.23243494969264E-7));
#12351=CARTESIAN_POINT('Ctrl Pts',(0.138491701959641,1.40582727297256,5.92673833856784E-7));
#12352=CARTESIAN_POINT('Ctrl Pts',(0.135853645420207,1.40411450883245,9.74556207071009E-7));
#12353=CARTESIAN_POINT('Ctrl Pts',(0.120686164410185,1.39426698768136,3.17018528370531E-6));
#12354=CARTESIAN_POINT('Ctrl Pts',(0.106484701177391,1.38310949089167,6.09567884445769E-6));
#12355=CARTESIAN_POINT('Ctrl Pts',(0.0934509959242968,1.37075049507673,
5.10227143121889E-6));
#12356=CARTESIAN_POINT('Ctrl Pts',(0.0918301157095608,1.36921352217444,
4.97873062758527E-6));
#12357=CARTESIAN_POINT('Ctrl Pts',(0.0902273306836925,1.36765791150105,
4.78983320752683E-6));
#12358=CARTESIAN_POINT('Ctrl Pts',(0.0886430622088043,1.36608382581751,
4.52250464763623E-6));
#12359=CARTESIAN_POINT('Ctrl Pts',(0.0755027622673366,1.35302798437193,
2.30521792157715E-6));
#12360=CARTESIAN_POINT('Ctrl Pts',(0.0636322991078783,1.33870385142449,
-4.95851449924696E-6));
#12361=CARTESIAN_POINT('Ctrl Pts',(0.0531272107863483,1.3233265665666,-1.07771754856876E-5));
#12362=CARTESIAN_POINT('Ctrl Pts',(0.0429100363670196,1.3083707283404,-1.64363639061758E-5));
#12363=CARTESIAN_POINT('Ctrl Pts',(0.0340657397255946,1.29253754778979,
-2.07072841115287E-5));
#12364=CARTESIAN_POINT('Ctrl Pts',(0.026663056477648,1.27603964904139,-2.15377272154938E-5));
#12365=CARTESIAN_POINT('Ctrl Pts',(0.0217318501145713,1.26504977678014,
-2.20909166714363E-5));
#12366=CARTESIAN_POINT('Ctrl Pts',(0.0174411483101006,1.25376411673155,
-2.12025196266096E-5));
#12367=CARTESIAN_POINT('Ctrl Pts',(0.01382286588119,1.24224013948332,-1.91534441809703E-5));
#12368=CARTESIAN_POINT('Ctrl Pts',(0.00842668188255806,1.22505366970124,
-1.60975223868617E-5));
#12369=CARTESIAN_POINT('Ctrl Pts',(0.00456091079961661,1.20745571355567,
-1.03588883906395E-5));
#12370=CARTESIAN_POINT('Ctrl Pts',(0.0023097402764219,1.18964331095195,
-5.71664032024866E-6));
#12371=CARTESIAN_POINT('Ctrl Pts',(0.00078319128522165,1.17756448131848,
-2.56866950429304E-6));
#12372=CARTESIAN_POINT('Ctrl Pts',(2.50028438421117E-9,1.16538650529032,
-1.91718613723104E-10));
#12373=CARTESIAN_POINT('Ctrl Pts',(-1.21430643318376E-17,1.15316892111333,
5.20417042793042E-18));
#12374=CARTESIAN_POINT('',(11.7295909468525,1.62672708026858,5.55111512312578E-17));
#12375=CARTESIAN_POINT('Ctrl Pts',(0.243580684154574,1.44748675362873,0.));
#12376=CARTESIAN_POINT('Ctrl Pts',(4.07225077172054,2.17467835246083,0.));
#12377=CARTESIAN_POINT('Ctrl Pts',(7.90092085928651,2.00057770191527,0.));
#12378=CARTESIAN_POINT('Ctrl Pts',(11.7295909468525,1.62672708026858,0.));
#12379=CARTESIAN_POINT('',(12.,1.32855945177638,-4.17473993839455E-17));
#12380=CARTESIAN_POINT('Ctrl Pts',(12.,1.32855945177638,2.42861286636753E-16));
#12381=CARTESIAN_POINT('Ctrl Pts',(11.9999999991614,1.34640852075174,-1.28298622986823E-11));
#12382=CARTESIAN_POINT('Ctrl Pts',(11.9983618543561,1.36418409382152,-2.22383001277967E-6));
#12383=CARTESIAN_POINT('Ctrl Pts',(11.9951861391139,1.38167870884165,-3.43465861540838E-6));
#12384=CARTESIAN_POINT('Ctrl Pts',(11.9919727904737,1.39938064150867,-4.65983598400874E-6));
#12385=CARTESIAN_POINT('Ctrl Pts',(11.9871848331028,1.41679645887758,-4.78742071954366E-6));
#12386=CARTESIAN_POINT('Ctrl Pts',(11.9808755917115,1.43370272794343,-3.5739118077222E-6));
#12387=CARTESIAN_POINT('Ctrl Pts',(11.9797611226834,1.43668906371449,-3.35955670324834E-6));
#12388=CARTESIAN_POINT('Ctrl Pts',(11.9785990681726,1.43965944485564,-3.11247275469786E-6));
#12389=CARTESIAN_POINT('Ctrl Pts',(11.9773895732386,1.44261255525912,-2.84353511336506E-6));
#12390=CARTESIAN_POINT('Ctrl Pts',(11.9705369081732,1.45934406518776,-1.31980853313606E-6));
#12391=CARTESIAN_POINT('Ctrl Pts',(11.9622259501015,1.47537448669426,1.24030492427686E-6));
#12392=CARTESIAN_POINT('Ctrl Pts',(11.9525330320198,1.49048867890869,8.79804099270529E-7));
#12393=CARTESIAN_POINT('Ctrl Pts',(11.9492586078121,1.49559449703792,7.58021100761347E-7));
#12394=CARTESIAN_POINT('Ctrl Pts',(11.9458260650319,1.50059560584699,2.73671093112169E-7));
#12395=CARTESIAN_POINT('Ctrl Pts',(11.9422371454499,1.50548309160802,-8.21070286398525E-7));
#12396=CARTESIAN_POINT('Ctrl Pts',(11.9335276940755,1.51734385321214,-3.47774636801117E-6));
#12397=CARTESIAN_POINT('Ctrl Pts',(11.923898315087,1.52853671512454,-9.61160164537397E-6));
#12398=CARTESIAN_POINT('Ctrl Pts',(11.9134480753511,1.53899918600446,-1.54908303532852E-5));
#12399=CARTESIAN_POINT('Ctrl Pts',(11.9006414429521,1.55182080751067,-2.26957483986032E-5));
#12400=CARTESIAN_POINT('Ctrl Pts',(11.8867118754531,1.56343792791748,-2.93307907620841E-5));
#12401=CARTESIAN_POINT('Ctrl Pts',(11.8718669715436,1.57375979462261,-3.2097080434168E-5));
#12402=CARTESIAN_POINT('Ctrl Pts',(11.8583226919989,1.58317731924447,-3.46210038525051E-5));
#12403=CARTESIAN_POINT('Ctrl Pts',(11.84401509256,1.59151672629289,-3.39892197405707E-5));
#12404=CARTESIAN_POINT('Ctrl Pts',(11.8290799708805,1.59867837245092,-3.04453078860132E-5));
#12405=CARTESIAN_POINT('Ctrl Pts',(11.8128282236205,1.60647136308226,-2.65889777530425E-5));
#12406=CARTESIAN_POINT('Ctrl Pts',(11.7959622791259,1.61280865470064,-1.93051308245346E-5));
#12407=CARTESIAN_POINT('Ctrl Pts',(11.7786680578171,1.61758555622507,-1.24065785496921E-5));
#12408=CARTESIAN_POINT('Ctrl Pts',(11.7626326571209,1.62201475420184,-6.0101616208217E-6));
#12409=CARTESIAN_POINT('Ctrl Pts',(11.7462278952123,1.62510256303752,-1.15598952599692E-10));
#12410=CARTESIAN_POINT('Ctrl Pts',(11.7295909468525,1.62672708026857,-1.01481323344643E-16));
#12411=CARTESIAN_POINT('',(12.,-1.32855945177638,-2.7831599589297E-17));
#12412=CARTESIAN_POINT('',(12.,1.6,0.));
#12413=CARTESIAN_POINT('',(11.7295909468525,-1.62672708026858,-2.77555756156289E-17));
#12414=CARTESIAN_POINT('Ctrl Pts',(11.7295909468525,-1.62672708026858,2.76688394418301E-16));
#12415=CARTESIAN_POINT('Ctrl Pts',(11.7473502233519,-1.62499297457843,3.63491969896433E-13));
#12416=CARTESIAN_POINT('Ctrl Pts',(11.7648769397846,-1.62163540491215,-2.46542030701863E-6));
#12417=CARTESIAN_POINT('Ctrl Pts',(11.7819744899096,-1.61677476461769,-3.87870576098494E-6));
#12418=CARTESIAN_POINT('Ctrl Pts',(11.799277951102,-1.61185558613358,-5.30901184740094E-6));
#12419=CARTESIAN_POINT('Ctrl Pts',(11.8161433440738,-1.60539638769883,-5.61072687595782E-6));
#12420=CARTESIAN_POINT('Ctrl Pts',(11.8323535184498,-1.59747214364331,-4.43708131311936E-6));
#12421=CARTESIAN_POINT('Ctrl Pts',(11.8351986841263,-1.59608130189932,-4.23108623901291E-6));
#12422=CARTESIAN_POINT('Ctrl Pts',(11.8380235988884,-1.59464521634493,-3.98890160078043E-6));
#12423=CARTESIAN_POINT('Ctrl Pts',(11.8408269920241,-1.59316415515964,-3.72087260345577E-6));
#12424=CARTESIAN_POINT('Ctrl Pts',(11.8568148563263,-1.58471760338924,-2.19229240409177E-6));
#12425=CARTESIAN_POINT('Ctrl Pts',(11.8719627312575,-1.57488689795395,5.08047814114288E-7));
#12426=CARTESIAN_POINT('Ctrl Pts',(11.8860639991294,-1.56376935451958,3.7910357452838E-7));
#12427=CARTESIAN_POINT('Ctrl Pts',(11.8908390360804,-1.5600046802233,3.35439876042474E-7));
#12428=CARTESIAN_POINT('Ctrl Pts',(11.8954938739134,-1.55609205312677,-6.31409548673105E-8));
#12429=CARTESIAN_POINT('Ctrl Pts',(11.9000197537765,-1.55203410647271,-1.07033715310124E-6));
#12430=CARTESIAN_POINT('Ctrl Pts',(11.9109521284419,-1.54223203603875,-3.50324446252274E-6));
#12431=CARTESIAN_POINT('Ctrl Pts',(11.9211333865357,-1.53158293117673,-9.37257606292525E-6));
#12432=CARTESIAN_POINT('Ctrl Pts',(11.9305114837192,-1.52019095639426,-1.50133174764804E-5));
#12433=CARTESIAN_POINT('Ctrl Pts',(11.9420285825687,-1.50620064502377,-2.19406264148308E-5));
#12434=CARTESIAN_POINT('Ctrl Pts',(11.9522379825693,-1.49120969914507,-2.8349487615449E-5));
#12435=CARTESIAN_POINT('Ctrl Pts',(11.9610699533786,-1.47543375940277,-3.10096306454085E-5));
#12436=CARTESIAN_POINT('Ctrl Pts',(11.9691383866925,-1.46102167397773,-3.34398002084833E-5));
#12437=CARTESIAN_POINT('Ctrl Pts',(11.976057247492,-1.44595309822982,-3.28127654573608E-5));
#12438=CARTESIAN_POINT('Ctrl Pts',(11.9817405815488,-1.43037347552767,-2.93737351251587E-5));
#12439=CARTESIAN_POINT('Ctrl Pts',(11.9879190063177,-1.41343666945002,-2.56351214921306E-5));
#12440=CARTESIAN_POINT('Ctrl Pts',(11.9925890154887,-1.39602986621001,-1.86015881889918E-5));
#12441=CARTESIAN_POINT('Ctrl Pts',(11.9956646601292,-1.37834843064327,-1.1951505214167E-5));
#12442=CARTESIAN_POINT('Ctrl Pts',(11.9985188379205,-1.36194017591583,-5.78027239782095E-6));
#12443=CARTESIAN_POINT('Ctrl Pts',(11.9999999979315,-1.34529424449622,-1.63143103698095E-10));
#12444=CARTESIAN_POINT('Ctrl Pts',(12.,-1.32855945177638,6.07153216591882E-17));
#12445=CARTESIAN_POINT('',(0.243580684154574,-1.44748675362873,-2.77555756156289E-17));
#12446=CARTESIAN_POINT('Ctrl Pts',(11.7295909468525,-1.62672708026858,0.));
#12447=CARTESIAN_POINT('Ctrl Pts',(7.90092085928651,-2.00057770191527,0.));
#12448=CARTESIAN_POINT('Ctrl Pts',(4.07225077172054,-2.17467835246083,0.));
#12449=CARTESIAN_POINT('Ctrl Pts',(0.243580684154574,-1.44748675362873,
0.));
#12450=CARTESIAN_POINT('',(-2.01407162049393E-18,-1.15316892111334,-2.77409355997279E-17));
#12451=CARTESIAN_POINT('Ctrl Pts',(-1.45716771982052E-16,-1.15316892111333,
-8.67361737988404E-17));
#12452=CARTESIAN_POINT('Ctrl Pts',(1.25998894435939E-9,-1.17105087373522,
-1.90287520688926E-11));
#12453=CARTESIAN_POINT('Ctrl Pts',(0.00163339464743996,-1.18886359576077,
-1.42965894531121E-6));
#12454=CARTESIAN_POINT('Ctrl Pts',(0.00480727841906161,-1.20639511031145,
-1.64093682142839E-6));
#12455=CARTESIAN_POINT('Ctrl Pts',(0.00800796397580062,-1.22407466931478,
-1.8539988284852E-6));
#12456=CARTESIAN_POINT('Ctrl Pts',(0.0127756311263789,-1.24146980201313,
-7.66483898132055E-7));
#12457=CARTESIAN_POINT('Ctrl Pts',(0.0190655400899108,-1.25835467436912,
1.24978183846727E-6));
#12458=CARTESIAN_POINT('Ctrl Pts',(0.0201762582672253,-1.26133632875492,
1.60582880463507E-6));
#12459=CARTESIAN_POINT('Ctrl Pts',(0.0213345630164365,-1.2643020159517,
1.98173645466097E-6));
#12460=CARTESIAN_POINT('Ctrl Pts',(0.022540357064946,-1.26725040777374,
2.36324320385681E-6));
#12461=CARTESIAN_POINT('Ctrl Pts',(0.0293845669280623,-1.28398578013164,
4.5287143794027E-6));
#12462=CARTESIAN_POINT('Ctrl Pts',(0.0376942987862453,-1.30001720705818,
7.20349268724091E-6));
#12463=CARTESIAN_POINT('Ctrl Pts',(0.0474014865253391,-1.31512615530125,
5.82569015349308E-6));
#12464=CARTESIAN_POINT('Ctrl Pts',(0.0485928463173857,-1.31698047129067,
5.65659292531477E-6));
#12465=CARTESIAN_POINT('Ctrl Pts',(0.049805315173965,-1.3188208685659,5.4220814195758E-6));
#12466=CARTESIAN_POINT('Ctrl Pts',(0.0510388164126442,-1.32064691964073,
5.10992468070797E-6));
#12467=CARTESIAN_POINT('Ctrl Pts',(0.0614399911345998,-1.33604461498541,
2.47774509321499E-6));
#12468=CARTESIAN_POINT('Ctrl Pts',(0.0733332132114129,-1.35042574344132,
-5.3152380038924E-6));
#12469=CARTESIAN_POINT('Ctrl Pts',(0.0865238753361435,-1.36365441213776,
-1.1550981620978E-5));
#12470=CARTESIAN_POINT('Ctrl Pts',(0.0993129767592984,-1.37648036310613,
-1.75968917362996E-5));
#12471=CARTESIAN_POINT('Ctrl Pts',(0.113220041589059,-1.38812080263946,
-2.21381304374214E-5));
#12472=CARTESIAN_POINT('Ctrl Pts',(0.128049501721596,-1.3984678073416,-2.30260298918279E-5));
#12473=CARTESIAN_POINT('Ctrl Pts',(0.137898881094142,-1.40534004502052,
-2.36157518704412E-5));
#12474=CARTESIAN_POINT('Ctrl Pts',(0.148156110210342,-1.41164106947418,
-2.26770903305374E-5));
#12475=CARTESIAN_POINT('Ctrl Pts',(0.158771208267938,-1.41732893485082,
-2.05010084084185E-5));
#12476=CARTESIAN_POINT('Ctrl Pts',(0.174640735071984,-1.42583226958806,
-1.72477751171679E-5));
#12477=CARTESIAN_POINT('Ctrl Pts',(0.191199787345415,-1.4329086754137,-1.11085100333009E-5));
#12478=CARTESIAN_POINT('Ctrl Pts',(0.208270835533445,-1.43843835369108,
-6.12965879291162E-6));
#12479=CARTESIAN_POINT('Ctrl Pts',(0.219822542278978,-1.44218019901621,
-2.76054936125183E-6));
#12480=CARTESIAN_POINT('Ctrl Pts',(0.231609382520684,-1.4452130041726,-1.10646384277296E-10));
#12481=CARTESIAN_POINT('Ctrl Pts',(0.243580684154575,-1.44748675362873,
-8.67361737988404E-18));
#12482=CARTESIAN_POINT('',(0.,-1.4,0.));
#12483=CARTESIAN_POINT('',(0.28146619846596,-1.25073018526678,-1.38777878078145E-17));
#12484=CARTESIAN_POINT('Ctrl Pts',(0.200274469199584,-1.15262458915154,
-4.38017677684144E-17));
#12485=CARTESIAN_POINT('Ctrl Pts',(0.200274469606231,-1.16056122076396,
-2.67994619525583E-11));
#12486=CARTESIAN_POINT('Ctrl Pts',(0.201251993787099,-1.16844573575355,
-2.06906772440415E-6));
#12487=CARTESIAN_POINT('Ctrl Pts',(0.203125250303271,-1.17612349127761,
-3.03593176598444E-6));
#12488=CARTESIAN_POINT('Ctrl Pts',(0.204328175564463,-1.18105381768481,
-3.65681052429326E-6));
#12489=CARTESIAN_POINT('Ctrl Pts',(0.205901645655995,-1.18589907428975,
-3.87486521964464E-6));
#12490=CARTESIAN_POINT('Ctrl Pts',(0.207834893326199,-1.19061551412018,
-3.56660141708203E-6));
#12491=CARTESIAN_POINT('Ctrl Pts',(0.210845733886816,-1.19796089907112,
-3.08651126907409E-6));
#12492=CARTESIAN_POINT('Ctrl Pts',(0.214691665920849,-1.20490884791767,
-1.13290501265697E-6));
#12493=CARTESIAN_POINT('Ctrl Pts',(0.219311372289421,-1.21130241743461,
-1.88024479619773E-7));
#12494=CARTESIAN_POINT('Ctrl Pts',(0.220549822002528,-1.21301640393121,
6.52788543367939E-8));
#12495=CARTESIAN_POINT('Ctrl Pts',(0.22184414018537,-1.21469042595737,2.26073670777299E-7));
#12496=CARTESIAN_POINT('Ctrl Pts',(0.223193686901845,-1.21632111014354,
1.99977909429435E-7));
#12497=CARTESIAN_POINT('Ctrl Pts',(0.225054776233359,-1.21856990146355,
1.63990609064731E-7));
#12498=CARTESIAN_POINT('Ctrl Pts',(0.227020882846909,-1.2207363067163,-2.2494482424301E-7));
#12499=CARTESIAN_POINT('Ctrl Pts',(0.229085096241527,-1.22281561536867,
-7.25033596408456E-7));
#12500=CARTESIAN_POINT('Ctrl Pts',(0.234663732853057,-1.22843504764494,
-2.07654770860772E-6));
#12501=CARTESIAN_POINT('Ctrl Pts',(0.240898147116973,-1.23336261820331,
-3.93931381885212E-6));
#12502=CARTESIAN_POINT('Ctrl Pts',(0.247634917667946,-1.2375211924479,-4.15647360184107E-6));
#12503=CARTESIAN_POINT('Ctrl Pts',(0.24944409362824,-1.23863798757926,-4.21479238469909E-6));
#12504=CARTESIAN_POINT('Ctrl Pts',(0.251289686356224,-1.23969909864123,
-4.17584617698396E-6));
#12505=CARTESIAN_POINT('Ctrl Pts',(0.253169062337335,-1.24070249413235,
-4.04352721072409E-6));
#12506=CARTESIAN_POINT('Ctrl Pts',(0.260147540238377,-1.24442829106235,
-3.55220190316667E-6));
#12507=CARTESIAN_POINT('Ctrl Pts',(0.267526846148503,-1.24732811138375,
-1.51439637010182E-6));
#12508=CARTESIAN_POINT('Ctrl Pts',(0.275164162321015,-1.24931347733136,
-4.73394739174148E-7));
#12509=CARTESIAN_POINT('Ctrl Pts',(0.277246452424842,-1.24985478107889,
-1.89568936341825E-7));
#12510=CARTESIAN_POINT('Ctrl Pts',(0.27934803608603,-1.25032783487679,-4.20368826828312E-12));
#12511=CARTESIAN_POINT('Ctrl Pts',(0.28146619846596,-1.25073018526678,1.2793585635329E-17));
#12512=CARTESIAN_POINT('',(0.9,-1.3604297237941,0.));
#12513=CARTESIAN_POINT('Ctrl Pts',(0.281466198465954,-1.25073018526678,
9.63150999927498E-16));
#12514=CARTESIAN_POINT('Ctrl Pts',(0.487510152792939,-1.28986875705046,
1.95065110193295E-11));
#12515=CARTESIAN_POINT('Ctrl Pts',(0.693681940810289,-1.32640030557063,
-1.68784634270162E-7));
#12516=CARTESIAN_POINT('Ctrl Pts',(0.899999999999961,-1.36042972379409,
2.52314774976951E-14));
#12517=CARTESIAN_POINT('',(0.9,1.44962962962963,0.));
#12518=CARTESIAN_POINT('',(3.9,-1.68995649764597,0.));
#12519=CARTESIAN_POINT('Ctrl Pts',(1.1,-1.39262953588351,-2.05019623674552E-17));
#12520=CARTESIAN_POINT('Ctrl Pts',(2.02971449277185,-1.53866936499954,-2.04062575199768E-17));
#12521=CARTESIAN_POINT('Ctrl Pts',(2.96251993741879,-1.63464569625347,-2.05230086706555E-17));
#12522=CARTESIAN_POINT('Ctrl Pts',(3.9,-1.68995649764597,-2.05203881127908E-17));
#12523=CARTESIAN_POINT('',(3.9,1.7662962962963,0.));
#12524=CARTESIAN_POINT('',(7.9,-1.70758761671949,0.));
#12525=CARTESIAN_POINT('Ctrl Pts',(4.10000000045307,-1.7011388979176,-4.27317380631109E-11));
#12526=CARTESIAN_POINT('Ctrl Pts',(4.72643887491804,-1.7342420350347,1.20853286712337E-7));
#12527=CARTESIAN_POINT('Ctrl Pts',(5.35502164560988,-1.74950180199062,-3.33551248611792E-7));
#12528=CARTESIAN_POINT('Ctrl Pts',(5.98619394951577,-1.74972093772735,-3.1920111515717E-7));
#12529=CARTESIAN_POINT('Ctrl Pts',(6.62418968669829,-1.74994244248134,-3.0469584628258E-7));
#12530=CARTESIAN_POINT('Ctrl Pts',(7.26228442347589,-1.73479337602516,3.6583895104054E-8));
#12531=CARTESIAN_POINT('Ctrl Pts',(7.90000000036908,-1.70758761645525,-3.06816097140251E-11));
#12532=CARTESIAN_POINT('',(7.9,1.7737037037037,0.));
#12533=CARTESIAN_POINT('',(11.4,-1.45718524058191,0.));
#12534=CARTESIAN_POINT('',(11.7095901160181,-1.42740242188993,1.38777878078145E-17));
#12535=CARTESIAN_POINT('Ctrl Pts',(11.4000000008084,-1.45718524050535,1.02728155843002E-16));
#12536=CARTESIAN_POINT('Ctrl Pts',(11.5032315878449,-1.44740895658952,-1.62414911853346E-10));
#12537=CARTESIAN_POINT('Ctrl Pts',(11.6064290066394,-1.43747657129068,3.17212713797596E-13));
#12538=CARTESIAN_POINT('Ctrl Pts',(11.7095901160181,-1.42740242188993,-1.31135713082882E-16));
#12539=CARTESIAN_POINT('',(11.7997255308004,-1.32801330383774,0.));
#12540=CARTESIAN_POINT('Ctrl Pts',(11.7095901160181,-1.42740242188993,-9.19403442267708E-17));
#12541=CARTESIAN_POINT('Ctrl Pts',(11.7174875668098,-1.42663119997609,-1.06723531187443E-12));
#12542=CARTESIAN_POINT('Ctrl Pts',(11.7252481284326,-1.42489860698852,-1.31351091787008E-6));
#12543=CARTESIAN_POINT('Ctrl Pts',(11.7327147629935,-1.4222933789697,-1.57347087725304E-6));
#12544=CARTESIAN_POINT('Ctrl Pts',(11.7375034508718,-1.42062252930751,-1.7401948673154E-6));
#12545=CARTESIAN_POINT('Ctrl Pts',(11.742171336984,-1.41859157258352,-1.52962160850981E-6));
#12546=CARTESIAN_POINT('Ctrl Pts',(11.7466731630754,-1.4162133745499,-1.06822103866601E-6));
#12547=CARTESIAN_POINT('Ctrl Pts',(11.7538080604269,-1.41244419322064,-3.36952074275293E-7));
#12548=CARTESIAN_POINT('Ctrl Pts',(11.7604421378066,-1.40785009750528,1.23525126371337E-6));
#12549=CARTESIAN_POINT('Ctrl Pts',(11.7664060685299,-1.40250292630552,-7.85770423176645E-8));
#12550=CARTESIAN_POINT('Ctrl Pts',(11.7700505374369,-1.39923534992309,-8.81437879006801E-7));
#12551=CARTESIAN_POINT('Ctrl Pts',(11.7734443324447,-1.39568546479044,-2.84121358692309E-6));
#12552=CARTESIAN_POINT('Ctrl Pts',(11.7765701913309,-1.39188797822873,-4.73246891796253E-6));
#12553=CARTESIAN_POINT('Ctrl Pts',(11.7816218974528,-1.38575085342217,-7.78893003218221E-6));
#12554=CARTESIAN_POINT('Ctrl Pts',(11.7859196635778,-1.3790373064984,-1.04294718165207E-5));
#12555=CARTESIAN_POINT('Ctrl Pts',(11.7894058487846,-1.37190723377291,-1.0649753115785E-5));
#12556=CARTESIAN_POINT('Ctrl Pts',(11.7909886780302,-1.36866997385604,-1.07497672177443E-5));
#12557=CARTESIAN_POINT('Ctrl Pts',(11.7924036476919,-1.36534638272796,-1.04045251440782E-5));
#12558=CARTESIAN_POINT('Ctrl Pts',(11.7936422141268,-1.36194984358789,-9.67400732978531E-6));
#12559=CARTESIAN_POINT('Ctrl Pts',(11.7963517531347,-1.35451943450186,-8.0758964348484E-6));
#12560=CARTESIAN_POINT('Ctrl Pts',(11.7981920551596,-1.34681816044402,-4.45435127417515E-6));
#12561=CARTESIAN_POINT('Ctrl Pts',(11.7990923524223,-1.33899256731255,-1.99131993767782E-6));
#12562=CARTESIAN_POINT('Ctrl Pts',(11.7995108157868,-1.33535518645399,-8.46488755312323E-7));
#12563=CARTESIAN_POINT('Ctrl Pts',(11.7997255306472,-1.33169069466208,-1.20180646731727E-11));
#12564=CARTESIAN_POINT('Ctrl Pts',(11.7997255308004,-1.32801330383774,1.56125112837913E-17));
#12565=CARTESIAN_POINT('',(11.7997255308004,1.32801330383774,-1.38777878078145E-17));
#12566=CARTESIAN_POINT('',(11.7997255308004,0.8,0.));
#12567=CARTESIAN_POINT('',(11.7095901160181,1.42740242188993,1.38777878078145E-17));
#12568=CARTESIAN_POINT('Ctrl Pts',(11.7997255308004,1.32801330383774,3.29597460435593E-17));
#12569=CARTESIAN_POINT('Ctrl Pts',(11.7997255306701,1.33594993357028,-3.19998942079111E-12));
#12570=CARTESIAN_POINT('Ctrl Pts',(11.7987557313351,1.34384388324515,-1.1738056914779E-6));
#12571=CARTESIAN_POINT('Ctrl Pts',(11.7968890528831,1.35153020534854,-1.35082478761126E-6));
#12572=CARTESIAN_POINT('Ctrl Pts',(11.7956902940742,1.35646627043222,-1.46450435604653E-6));
#12573=CARTESIAN_POINT('Ctrl Pts',(11.7941204989552,1.36131691981906,-1.21679535622301E-6));
#12574=CARTESIAN_POINT('Ctrl Pts',(11.7921880664813,1.36603565236267,-7.51718013047842E-7));
#12575=CARTESIAN_POINT('Ctrl Pts',(11.7891321441143,1.37349779167052,-1.62510435539431E-8));
#12576=CARTESIAN_POINT('Ctrl Pts',(11.7852081688769,1.38054242009704,1.47305143123643E-6));
#12577=CARTESIAN_POINT('Ctrl Pts',(11.7804707482717,1.38699431162271,4.31295153147674E-8));
#12578=CARTESIAN_POINT('Ctrl Pts',(11.7775673564694,1.39094843993989,-8.33217322910001E-7));
#12579=CARTESIAN_POINT('Ctrl Pts',(11.774357304366,1.39467961749964,-2.88177890715362E-6));
#12580=CARTESIAN_POINT('Ctrl Pts',(11.7708736118052,1.39816709864095,-4.85419454747415E-6));
#12581=CARTESIAN_POINT('Ctrl Pts',(11.7652557092992,1.40379111072049,-8.03496856102318E-6));
#12582=CARTESIAN_POINT('Ctrl Pts',(11.7589908599241,1.40872063947841,-1.07717451179728E-5));
#12583=CARTESIAN_POINT('Ctrl Pts',(11.7522324303862,1.41288246393566,-1.10093962897399E-5));
#12584=CARTESIAN_POINT('Ctrl Pts',(11.7491699691574,1.41476832010531,-1.11170836593312E-5));
#12585=CARTESIAN_POINT('Ctrl Pts',(11.7460056456443,1.41649603445901,-1.07652933077188E-5));
#12586=CARTESIAN_POINT('Ctrl Pts',(11.7427518690514,1.41805582819498,-1.00150721194158E-5));
#12587=CARTESIAN_POINT('Ctrl Pts',(11.7356218627913,1.421473806899,-8.37111113549047E-6));
#12588=CARTESIAN_POINT('Ctrl Pts',(11.7281378774234,1.42405291512428,-4.62166314666036E-6));
#12589=CARTESIAN_POINT('Ctrl Pts',(11.7204387731059,1.42570834923663,-2.06587013620581E-6));
#12590=CARTESIAN_POINT('Ctrl Pts',(11.7168648812537,1.42647679479109,-8.79481766934018E-7));
#12591=CARTESIAN_POINT('Ctrl Pts',(11.7132443218769,1.42704557200794,-8.45784208685192E-12));
#12592=CARTESIAN_POINT('Ctrl Pts',(11.7095901160181,1.42740242188993,2.53703308361608E-17));
#12593=CARTESIAN_POINT('',(11.4,1.45718524058191,0.));
#12594=CARTESIAN_POINT('Ctrl Pts',(11.7095901160181,1.42740242188993,-2.09644042577228E-16));
#12595=CARTESIAN_POINT('Ctrl Pts',(11.6064290073882,1.43747657121756,3.16925904777201E-13));
#12596=CARTESIAN_POINT('Ctrl Pts',(11.5032315885351,1.44740895652415,-1.62368751268212E-10));
#12597=CARTESIAN_POINT('Ctrl Pts',(11.4000000008083,1.45718524050537,-7.57963810214684E-17));
#12598=CARTESIAN_POINT('',(11.4,-1.53779953703704,0.));
#12599=CARTESIAN_POINT('Origin',(10.,0.,0.));
#12600=CARTESIAN_POINT('',(9.6,-4.89858719658942E-17,0.7));
#12601=CARTESIAN_POINT('Origin',(10.,0.,0.7));
#12602=CARTESIAN_POINT('',(9.6,-4.89858719658942E-17,0.));
#12603=CARTESIAN_POINT('Origin',(2.,0.,0.));
#12604=CARTESIAN_POINT('',(1.6,-4.89858719658941E-17,0.7));
#12605=CARTESIAN_POINT('Origin',(2.,0.,0.7));
#12606=CARTESIAN_POINT('',(1.6,-4.89858719658941E-17,0.));
#12607=CARTESIAN_POINT('Origin',(11.4,-1.53779953703704,0.));
#12608=CARTESIAN_POINT('',(11.4,-1.4227102204299,0.605660349289938));
#12609=CARTESIAN_POINT('Ctrl Pts',(11.4,-1.45718524058191,0.));
#12610=CARTESIAN_POINT('Ctrl Pts',(11.4,-1.45144762186897,0.100853500740053));
#12611=CARTESIAN_POINT('Ctrl Pts',(11.4,-1.44570843451869,0.201707502489292));
#12612=CARTESIAN_POINT('Ctrl Pts',(11.4,-1.43421679834229,0.403593890565801));
#12613=CARTESIAN_POINT('Ctrl Pts',(11.4,-1.42846427656079,0.504627461196798));
#12614=CARTESIAN_POINT('Ctrl Pts',(11.4,-1.4227102204299,0.605660349289938));
#12615=CARTESIAN_POINT('',(11.4,1.4227102204299,0.605660349289938));
#12616=CARTESIAN_POINT('Ctrl Pts',(11.4,1.4227102204299,0.605660349289938));
#12617=CARTESIAN_POINT('Ctrl Pts',(11.4,1.42846501637408,0.504614471147338));
#12618=CARTESIAN_POINT('Ctrl Pts',(11.4,1.43421827757761,0.403567910233218));
#12619=CARTESIAN_POINT('Ctrl Pts',(11.4,1.44570991295315,0.201681522149997));
#12620=CARTESIAN_POINT('Ctrl Pts',(11.4,1.45144836088146,0.100840510682596));
#12621=CARTESIAN_POINT('Ctrl Pts',(11.4,1.45718524058191,0.));
#12622=CARTESIAN_POINT('',(11.4,1.32241589772268,0.7));
#12623=CARTESIAN_POINT('Ctrl Pts',(11.3999999999682,1.32241589773435,0.7));
#12624=CARTESIAN_POINT('Ctrl Pts',(11.4000000023735,1.33035873561384,0.69999999792071));
#12625=CARTESIAN_POINT('Ctrl Pts',(11.3999980827719,1.33823923135401,0.699006238562837));
#12626=CARTESIAN_POINT('Ctrl Pts',(11.3999964146773,1.34591623266897,0.697118452648154));
#12627=CARTESIAN_POINT('Ctrl Pts',(11.3999954805754,1.35021521026861,0.696061327733467));
#12628=CARTESIAN_POINT('Ctrl Pts',(11.3999946303028,1.35445042327231,0.694722827332644));
#12629=CARTESIAN_POINT('Ctrl Pts',(11.3999940855437,1.35859537550353,0.6931136259882));
#12630=CARTESIAN_POINT('Ctrl Pts',(11.3999931076272,1.36603612757745,0.690224891070856));
#12631=CARTESIAN_POINT('Ctrl Pts',(11.3999932937992,1.3731074395729,0.686497549823264));
#12632=CARTESIAN_POINT('Ctrl Pts',(11.3999945206258,1.37966241828116,0.682010734965951));
#12633=CARTESIAN_POINT('Ctrl Pts',(11.3999951957832,1.38326980879772,0.679541513617388));
#12634=CARTESIAN_POINT('Ctrl Pts',(11.399996159718,1.38672054258633,0.67684140394947));
#12635=CARTESIAN_POINT('Ctrl Pts',(11.3999970106794,1.38998612808193,0.67391813047908));
#12636=CARTESIAN_POINT('Ctrl Pts',(11.399997834674,1.39314822810011,0.671087494715186));
#12637=CARTESIAN_POINT('Ctrl Pts',(11.3999985616145,1.39611771109305,0.668064564866167));
#12638=CARTESIAN_POINT('Ctrl Pts',(11.3999985600482,1.39887227052748,0.664860274403491));
#12639=CARTESIAN_POINT('Ctrl Pts',(11.3999985571253,1.40401282028653,0.65888043807832));
#12640=CARTESIAN_POINT('Ctrl Pts',(11.3999962993541,1.40840780441339,0.652270325570232));
#12641=CARTESIAN_POINT('Ctrl Pts',(11.399995545677,1.411994629421,0.6451936465425));
#12642=CARTESIAN_POINT('Ctrl Pts',(11.3999954685939,1.41236147527551,0.644469872631166));
#12643=CARTESIAN_POINT('Ctrl Pts',(11.3999954033687,1.41271982702329,0.643741199273148));
#12644=CARTESIAN_POINT('Ctrl Pts',(11.399995351278,1.41306958904162,0.643007791034547));
#12645=CARTESIAN_POINT('Ctrl Pts',(11.3999948427782,1.41648390439843,0.635848388696429));
#12646=CARTESIAN_POINT('Ctrl Pts',(11.3999960181446,1.41904356023948,0.628323447569199));
#12647=CARTESIAN_POINT('Ctrl Pts',(11.3999977140636,1.42069349507095,0.620600117586001));
#12648=CARTESIAN_POINT('Ctrl Pts',(11.3999987928026,1.4217429844709,0.615687467222433));
#12649=CARTESIAN_POINT('Ctrl Pts',(11.4,1.42242354791745,0.610693903223035));
#12650=CARTESIAN_POINT('Ctrl Pts',(11.4,1.42271022042989,0.605660349289938));
#12651=CARTESIAN_POINT('',(11.4,-1.32241589772233,0.7));
#12652=CARTESIAN_POINT('',(11.4,-0.768899768518519,0.7));
#12653=CARTESIAN_POINT('Ctrl Pts',(11.4,-1.4227102204299,0.605660349289938));
#12654=CARTESIAN_POINT('Ctrl Pts',(11.4,-1.42225988230954,0.613567634148305));
#12655=CARTESIAN_POINT('Ctrl Pts',(11.399997277834,-1.42084002197897,0.621378952482038));
#12656=CARTESIAN_POINT('Ctrl Pts',(11.3999960666067,-1.41853584574224,0.62893480307212));
#12657=CARTESIAN_POINT('Ctrl Pts',(11.3999954054252,-1.41727804822547,0.633059370437125));
#12658=CARTESIAN_POINT('Ctrl Pts',(11.399995101512,-1.41575577202439,0.637107840337094));
#12659=CARTESIAN_POINT('Ctrl Pts',(11.3999952458732,-1.4139766528271,0.641052464558972));
#12660=CARTESIAN_POINT('Ctrl Pts',(11.3999955106959,-1.41071295596475,0.648288661951321));
#12661=CARTESIAN_POINT('Ctrl Pts',(11.3999975070228,-1.40662392062869,0.655096264526915));
#12662=CARTESIAN_POINT('Ctrl Pts',(11.3999983091255,-1.40177626405188,0.661313589686923));
#12663=CARTESIAN_POINT('Ctrl Pts',(11.3999984645713,-1.40083679843637,0.66251849418371));
#12664=CARTESIAN_POINT('Ctrl Pts',(11.3999985618942,-1.3998687022723,0.663701157110503));
#12665=CARTESIAN_POINT('Ctrl Pts',(11.3999985615247,-1.39887227038638,0.664860274403572));
#12666=CARTESIAN_POINT('Ctrl Pts',(11.3999985608543,-1.39706426040285,0.666963474499402));
#12667=CARTESIAN_POINT('Ctrl Pts',(11.3999982409398,-1.39516298427334,0.668989190735049));
#12668=CARTESIAN_POINT('Ctrl Pts',(11.3999977953094,-1.39317470503404,0.670934323115149));
#12669=CARTESIAN_POINT('Ctrl Pts',(11.3999965209597,-1.38748891009577,0.67649673287249));
#12670=CARTESIAN_POINT('Ctrl Pts',(11.3999944455422,-1.38115857071774,0.681340422576046));
#12671=CARTESIAN_POINT('Ctrl Pts',(11.3999937508435,-1.37434881732181,0.685413525744465));
#12672=CARTESIAN_POINT('Ctrl Pts',(11.3999933041982,-1.36997059693002,0.688032261301096));
#12673=CARTESIAN_POINT('Ctrl Pts',(11.3999933336943,-1.3653932120823,0.69033179581025));
#12674=CARTESIAN_POINT('Ctrl Pts',(11.399993839827,-1.36065445462682,0.69228884175444));
#12675=CARTESIAN_POINT('Ctrl Pts',(11.3999946245508,-1.35330733883187,0.695323106179894));
#12676=CARTESIAN_POINT('Ctrl Pts',(11.3999965692242,-1.34565642326237,0.69750197024776));
#12677=CARTESIAN_POINT('Ctrl Pts',(11.3999981510416,-1.33784990929195,0.698756936804364));
#12678=CARTESIAN_POINT('Ctrl Pts',(11.399999182603,-1.33275899381189,0.699575346749464));
#12679=CARTESIAN_POINT('Ctrl Pts',(11.4000000015384,-1.32760128986121,0.699999998642559));
#12680=CARTESIAN_POINT('Ctrl Pts',(11.3999999999682,-1.32241589773435,0.7));
#12681=CARTESIAN_POINT('Ctrl Pts',(11.227882892666,-1.47337141465794,-0.000640335460849732));
#12682=CARTESIAN_POINT('Ctrl Pts',(11.218588765022,-1.46278323638644,0.201451598614313));
#12683=CARTESIAN_POINT('Ctrl Pts',(11.2092944683555,-1.45219508216535,0.40354352620373));
#12684=CARTESIAN_POINT('Ctrl Pts',(11.2000000000001,-1.44160695250309,0.60563544721184));
#12685=CARTESIAN_POINT('Ctrl Pts',(10.1843397214697,-1.57034855377304,-0.000384310983874139));
#12686=CARTESIAN_POINT('Ctrl Pts',(10.1768953195658,-1.55975965902304,0.201708049868595));
#12687=CARTESIAN_POINT('Ctrl Pts',(10.1694507716805,-1.54917076711515,0.403800406245857));
#12688=CARTESIAN_POINT('Ctrl Pts',(10.1620060668616,-1.53858190981164,0.605892758286982));
#12689=CARTESIAN_POINT('Ctrl Pts',(9.14170648965309,-1.65016851777514,-0.000148134864058495));
#12690=CARTESIAN_POINT('Ctrl Pts',(9.13611341817177,-1.63957870617509,0.201944615677573));
#12691=CARTESIAN_POINT('Ctrl Pts',(9.13052023035058,-1.6289888900612,0.404037363603497));
#12692=CARTESIAN_POINT('Ctrl Pts',(9.124926910836,-1.6183991014662,0.606130109186173));
#12693=CARTESIAN_POINT('Ctrl Pts',(8.1,-1.69866351109718,1.00613961606655E-16));
#12694=CARTESIAN_POINT('Ctrl Pts',(8.09625995443094,-1.68807302815665,0.202092993803311));
#12695=CARTESIAN_POINT('Ctrl Pts',(8.09251982249141,-1.67748255132318,0.404185986335255));
#12696=CARTESIAN_POINT('Ctrl Pts',(8.08877960280056,-1.66689208072706,0.606278977577217));
#12697=CARTESIAN_POINT('Ctrl Pts',(8.1,-1.66641703131627,0.605314487869832));
#12698=CARTESIAN_POINT('Ctrl Pts',(9.13548525483003,-1.617718421277,0.605389190939432));
#12699=CARTESIAN_POINT('Ctrl Pts',(10.168822041161,-1.53796707615457,0.605507632815633));
#12700=CARTESIAN_POINT('Ctrl Pts',(11.2000000000893,-1.44160695345912,0.605635447210802));
#12701=CARTESIAN_POINT('Ctrl Pts',(11.7095939787209,-1.42740645209206,-7.69249563980189E-5));
#12702=CARTESIAN_POINT('Ctrl Pts',(11.6994545874061,-1.41682738380082,0.201847033339061));
#12703=CARTESIAN_POINT('Ctrl Pts',(11.6893150192885,-1.40624834198077,0.403770984173611));
#12704=CARTESIAN_POINT('Ctrl Pts',(11.6791752715866,-1.39566932719028,0.605694927437301));
#12705=CARTESIAN_POINT('Ctrl Pts',(11.6063871276792,-1.43748358609578,-5.11721697277706E-5));
#12706=CARTESIAN_POINT('Ctrl Pts',(11.596430427176,-1.42690445239132,0.201872829148883));
#12707=CARTESIAN_POINT('Ctrl Pts',(11.5864735514701,-1.41632534465399,0.403796823219986));
#12708=CARTESIAN_POINT('Ctrl Pts',(11.5765164978042,-1.40574626343445,0.605720809936841));
#12709=CARTESIAN_POINT('Ctrl Pts',(11.5031891278894,-1.4474144288224,-2.55082377288765E-5));
#12710=CARTESIAN_POINT('Ctrl Pts',(11.4934151336386,-1.43683522760458,0.201898535909597));
#12711=CARTESIAN_POINT('Ctrl Pts',(11.4836409658656,-1.42625605183456,0.40382257302165));
#12712=CARTESIAN_POINT('Ctrl Pts',(11.4738666218385,-1.41567690205216,0.605746602994839));
#12713=CARTESIAN_POINT('Ctrl Pts',(11.4,-1.45718524058191,-5.20417042793042E-18));
#12714=CARTESIAN_POINT('Ctrl Pts',(11.3904087275488,-1.44660597001679,0.201924086674796));
#12715=CARTESIAN_POINT('Ctrl Pts',(11.3808172833376,-1.43602672436683,0.403848166524883));
#12716=CARTESIAN_POINT('Ctrl Pts',(11.3712256646606,-1.42544750415802,0.605772239449758));
#12717=CARTESIAN_POINT('',(11.6778970386953,-1.39579479040469,0.605695249702977));
#12718=CARTESIAN_POINT('Ctrl Pts',(11.4,-1.4227102204299,0.605660349289938));
#12719=CARTESIAN_POINT('Ctrl Pts',(11.4926474653491,-1.41386220753305,0.605671932550561));
#12720=CARTESIAN_POINT('Ctrl Pts',(11.585279512325,-1.40488700096013,0.605683574233495));
#12721=CARTESIAN_POINT('Ctrl Pts',(11.6778970386953,-1.39579479040469,0.605695249702977));
#12722=CARTESIAN_POINT('Ctrl Pts',(11.6778970386953,-1.39579479040469,0.605695249702977));
#12723=CARTESIAN_POINT('Ctrl Pts',(11.6884613130147,-1.40633044792991,0.403796817797553));
#12724=CARTESIAN_POINT('Ctrl Pts',(11.6990256725537,-1.41686632615463,0.201898401304098));
#12725=CARTESIAN_POINT('Ctrl Pts',(11.7095901160181,-1.42740242188993,5.19332840620557E-17));
#12726=CARTESIAN_POINT('Ctrl Pts',(11.2,-1.34133050917871,0.7));
#12727=CARTESIAN_POINT('Ctrl Pts',(10.1668086441106,-1.43797263608903,0.7));
#12728=CARTESIAN_POINT('Ctrl Pts',(9.13190264019122,-1.51792184128158,0.7));
#12729=CARTESIAN_POINT('Ctrl Pts',(8.09530923905977,-1.56666858280461,0.7));
#12730=CARTESIAN_POINT('Ctrl Pts',(11.2026864299662,-1.37005086445236,0.7));
#12731=CARTESIAN_POINT('Ctrl Pts',(10.1691860218014,-1.46674693471719,0.700000910790016));
#12732=CARTESIAN_POINT('Ctrl Pts',(9.13384227773975,-1.54675516497,0.699999464833944));
#12733=CARTESIAN_POINT('Ctrl Pts',(8.09666712422266,-1.59554384206015,0.700000000000001));
#12734=CARTESIAN_POINT('Ctrl Pts',(11.2073428085028,-1.4198317437391,0.676744232988519));
#12735=CARTESIAN_POINT('Ctrl Pts',(10.1733099382853,-1.51661799675652,0.676702307311825));
#12736=CARTESIAN_POINT('Ctrl Pts',(9.13719745543551,-1.59672983278297,0.676663906627884));
#12737=CARTESIAN_POINT('Ctrl Pts',(8.09902054834098,-1.64558911349573,0.676639354455264));
#12738=CARTESIAN_POINT('Ctrl Pts',(11.2091847227485,-1.43952346553595,0.627236497176141));
#12739=CARTESIAN_POINT('Ctrl Pts',(10.1749352046592,-1.53629892039422,0.62712791425818));
#12740=CARTESIAN_POINT('Ctrl Pts',(9.13852107143019,-1.61640633519008,0.627027713743691));
#12741=CARTESIAN_POINT('Ctrl Pts',(8.0999458765183,-1.66526610220338,0.626964226563296));
#12742=CARTESIAN_POINT('Ctrl Pts',(11.209298290232,-1.4407376041935,0.605636599993194));
#12743=CARTESIAN_POINT('Ctrl Pts',(10.1750338985877,-1.53748737250229,0.605508345221004));
#12744=CARTESIAN_POINT('Ctrl Pts',(9.13859765097935,-1.61757204607208,0.605389415477198));
#12745=CARTESIAN_POINT('Ctrl Pts',(8.1,-1.66641703131627,0.605314487869832));
#12746=CARTESIAN_POINT('Ctrl Pts',(11.2,-1.34133050917871,0.7));
#12747=CARTESIAN_POINT('Ctrl Pts',(10.16836710286,-1.43782686176815,0.7));
#12748=CARTESIAN_POINT('Ctrl Pts',(9.13502472651537,-1.51768061363633,0.7));
#12749=CARTESIAN_POINT('Ctrl Pts',(8.09999999865516,-1.56644778212326,0.7));
#12750=CARTESIAN_POINT('Ctrl Pts',(11.6681436286308,-1.2964346619681,0.7));
#12751=CARTESIAN_POINT('Ctrl Pts',(11.5756099286391,-1.3055179747114,0.7));
#12752=CARTESIAN_POINT('Ctrl Pts',(11.4830653488871,-1.31448403714215,0.7));
#12753=CARTESIAN_POINT('Ctrl Pts',(11.3905090053564,-1.32332268868375,0.7));
#12754=CARTESIAN_POINT('Ctrl Pts',(11.6709605510772,-1.32513126902304,0.700000000000001));
#12755=CARTESIAN_POINT('Ctrl Pts',(11.5784027531871,-1.33421922733773,0.700000082825348));
#12756=CARTESIAN_POINT('Ctrl Pts',(11.4858332859074,-1.34318985044544,0.699999917777441));
#12757=CARTESIAN_POINT('Ctrl Pts',(11.3932507170007,-1.35203326785046,0.7));
#12758=CARTESIAN_POINT('Ctrl Pts',(11.6758431636759,-1.37487151491717,0.67676311428296));
#12759=CARTESIAN_POINT('Ctrl Pts',(11.583243842395,-1.38396722707511,0.676759299309384));
#12760=CARTESIAN_POINT('Ctrl Pts',(11.4906306781253,-1.39294591144353,0.676755553516685));
#12761=CARTESIAN_POINT('Ctrl Pts',(11.3980029235659,-1.40179729139028,0.67675176769038));
#12762=CARTESIAN_POINT('Ctrl Pts',(11.6777767156198,-1.39456903283364,0.627286048421068));
#12763=CARTESIAN_POINT('Ctrl Pts',(11.5851604051362,-1.40366358810601,0.627276165220861));
#12764=CARTESIAN_POINT('Ctrl Pts',(11.4925297866457,-1.41264104586547,0.627266369072496));
#12765=CARTESIAN_POINT('Ctrl Pts',(11.3998836071583,-1.4214913811319,0.627256563056779));
#12766=CARTESIAN_POINT('Ctrl Pts',(11.6778970386953,-1.39579479040469,0.605695249702977));
#12767=CARTESIAN_POINT('Ctrl Pts',(11.585279512325,-1.40488700096013,0.605683574233495));
#12768=CARTESIAN_POINT('Ctrl Pts',(11.4926474653491,-1.41386220753305,0.605671932550561));
#12769=CARTESIAN_POINT('Ctrl Pts',(11.4,-1.4227102204299,0.605660349289938));
#12770=CARTESIAN_POINT('',(11.6681436286308,-1.2964346619681,0.7));
#12771=CARTESIAN_POINT('Ctrl Pts',(11.6681436286308,-1.2964346619681,0.7));
#12772=CARTESIAN_POINT('Ctrl Pts',(11.5787728332608,-1.30520749699507,0.7));
#12773=CARTESIAN_POINT('Ctrl Pts',(11.4893918891838,-1.31387096021207,0.7));
#12774=CARTESIAN_POINT('Ctrl Pts',(11.3999999999682,-1.32241589773435,0.7));
#12775=CARTESIAN_POINT('Origin',(11.6681436286308,-1.2964346619681,0.6));
#12776=CARTESIAN_POINT('Origin',(6.08012166120517,1.06778195214465E-16,
0.7));
#12777=CARTESIAN_POINT('Ctrl Pts',(8.0999999986552,1.56644778212326,0.7));
#12778=CARTESIAN_POINT('Ctrl Pts',(9.13502472651542,1.51768061363633,0.7));
#12779=CARTESIAN_POINT('Ctrl Pts',(10.16836710286,1.43782686176815,0.7));
#12780=CARTESIAN_POINT('Ctrl Pts',(11.2,1.34133050917871,0.7));
#12781=CARTESIAN_POINT('Origin',(6.08012166120517,1.06778195214465E-16,
0.7));
#12782=CARTESIAN_POINT('',(11.6681436286308,1.2964346619681,0.7));
#12783=CARTESIAN_POINT('Ctrl Pts',(11.3999999999682,1.32241589773435,0.7));
#12784=CARTESIAN_POINT('Ctrl Pts',(11.4893918891837,1.31387096021208,0.7));
#12785=CARTESIAN_POINT('Ctrl Pts',(11.5787728332608,1.30520749699508,0.7));
#12786=CARTESIAN_POINT('Ctrl Pts',(11.6681436286308,1.2964346619681,0.7));
#12787=CARTESIAN_POINT('',(11.6681436286308,0.8,0.7));
#12788=CARTESIAN_POINT('Ctrl Pts',(8.09530923905978,1.56666858280461,0.7));
#12789=CARTESIAN_POINT('Ctrl Pts',(9.13190264019124,1.51792184128158,0.7));
#12790=CARTESIAN_POINT('Ctrl Pts',(10.1668086441106,1.43797263608903,0.7));
#12791=CARTESIAN_POINT('Ctrl Pts',(11.2,1.34133050917871,0.7));
#12792=CARTESIAN_POINT('Ctrl Pts',(8.09666712422266,1.59554384206015,0.700000000000001));
#12793=CARTESIAN_POINT('Ctrl Pts',(9.13384227773977,1.54675516497,0.699999464833944));
#12794=CARTESIAN_POINT('Ctrl Pts',(10.1691860218013,1.46674693471719,0.700000910790016));
#12795=CARTESIAN_POINT('Ctrl Pts',(11.2026864299662,1.37005086445236,0.7));
#12796=CARTESIAN_POINT('Ctrl Pts',(8.09902054834099,1.64558911349573,0.676639354455264));
#12797=CARTESIAN_POINT('Ctrl Pts',(9.13719745543553,1.59672983278297,0.676663906627884));
#12798=CARTESIAN_POINT('Ctrl Pts',(10.1733099382853,1.51661799675652,0.676702307311825));
#12799=CARTESIAN_POINT('Ctrl Pts',(11.2073428085028,1.4198317437391,0.676744232988519));
#12800=CARTESIAN_POINT('Ctrl Pts',(8.0999458765183,1.66526610220338,0.626964226563296));
#12801=CARTESIAN_POINT('Ctrl Pts',(9.1385210714302,1.61640633519008,0.627027713743691));
#12802=CARTESIAN_POINT('Ctrl Pts',(10.1749352046592,1.53629892039423,0.62712791425818));
#12803=CARTESIAN_POINT('Ctrl Pts',(11.2091847227485,1.43952346553595,0.627236497176141));
#12804=CARTESIAN_POINT('Ctrl Pts',(8.1,1.66641703131627,0.605314487869832));
#12805=CARTESIAN_POINT('Ctrl Pts',(9.13859765097937,1.61757204607208,0.605389415477198));
#12806=CARTESIAN_POINT('Ctrl Pts',(10.1750338985877,1.53748737250229,0.605508345221004));
#12807=CARTESIAN_POINT('Ctrl Pts',(11.209298290232,1.4407376041935,0.605636599993194));
#12808=CARTESIAN_POINT('Ctrl Pts',(11.2000000000893,1.44160695345912,0.605635447210802));
#12809=CARTESIAN_POINT('Ctrl Pts',(10.168822041161,1.53796707615457,0.605507632815633));
#12810=CARTESIAN_POINT('Ctrl Pts',(9.13548525483005,1.617718421277,0.605389190939432));
#12811=CARTESIAN_POINT('Ctrl Pts',(8.1,1.66641703131627,0.605314487869832));
#12812=CARTESIAN_POINT('Ctrl Pts',(8.1,1.69866351109859,-2.6441702993818E-11));
#12813=CARTESIAN_POINT('Ctrl Pts',(8.09625995443078,1.68807302815759,0.202092993785684));
#12814=CARTESIAN_POINT('Ctrl Pts',(8.09251982249108,1.67748255132366,0.404185986326441));
#12815=CARTESIAN_POINT('Ctrl Pts',(8.08877960280008,1.66689208072708,0.606278977577217));
#12816=CARTESIAN_POINT('Ctrl Pts',(9.14170648965349,1.65016851777655,-0.00014813489050026));
#12817=CARTESIAN_POINT('Ctrl Pts',(9.13611341817193,1.63957870617604,0.201944615659945));
#12818=CARTESIAN_POINT('Ctrl Pts',(9.1305202303505,1.62898889006169,0.404037363594684));
#12819=CARTESIAN_POINT('Ctrl Pts',(9.12492691083567,1.61839910146622,0.606130109186173));
#12820=CARTESIAN_POINT('Ctrl Pts',(10.1843397214705,1.57034855377444,-0.000384311010315772));
#12821=CARTESIAN_POINT('Ctrl Pts',(10.1768953195662,1.55975965902398,0.201708049850968));
#12822=CARTESIAN_POINT('Ctrl Pts',(10.1694507716807,1.54917076711562,0.403800406237042));
#12823=CARTESIAN_POINT('Ctrl Pts',(10.1620060668615,1.53858190981166,0.605892758286982));
#12824=CARTESIAN_POINT('Ctrl Pts',(11.2278828926672,1.47337141465933,-0.000640335487291374));
#12825=CARTESIAN_POINT('Ctrl Pts',(11.2185887650228,1.46278323638736,0.201451598596686));
#12826=CARTESIAN_POINT('Ctrl Pts',(11.2092944683559,1.45219508216582,0.403543526194916));
#12827=CARTESIAN_POINT('Ctrl Pts',(11.2000000000001,1.44160695250309,0.60563544721184));
#12828=CARTESIAN_POINT('Ctrl Pts',(11.4,1.45718524058191,-1.37043154602168E-16));
#12829=CARTESIAN_POINT('Ctrl Pts',(11.3904087275488,1.44660597001679,0.201924086674796));
#12830=CARTESIAN_POINT('Ctrl Pts',(11.3808172833376,1.43602672436683,0.403848166524884));
#12831=CARTESIAN_POINT('Ctrl Pts',(11.3712256646606,1.42544750415802,0.605772239449759));
#12832=CARTESIAN_POINT('Ctrl Pts',(11.5031891278894,1.4474144288224,-2.55082377290153E-5));
#12833=CARTESIAN_POINT('Ctrl Pts',(11.4934151336386,1.43683522760458,0.201898535909598));
#12834=CARTESIAN_POINT('Ctrl Pts',(11.4836409658656,1.42625605183455,0.40382257302165));
#12835=CARTESIAN_POINT('Ctrl Pts',(11.4738666218385,1.41567690205216,0.605746602994839));
#12836=CARTESIAN_POINT('Ctrl Pts',(11.6063871276792,1.43748358609579,-5.1172169727805E-5));
#12837=CARTESIAN_POINT('Ctrl Pts',(11.596430427176,1.42690445239132,0.201872829148883));
#12838=CARTESIAN_POINT('Ctrl Pts',(11.5864735514701,1.41632534465399,0.403796823219986));
#12839=CARTESIAN_POINT('Ctrl Pts',(11.5765164978042,1.40574626343445,0.605720809936842));
#12840=CARTESIAN_POINT('Ctrl Pts',(11.7095939787209,1.42740645209206,-7.69249563980588E-5));
#12841=CARTESIAN_POINT('Ctrl Pts',(11.6994545874061,1.41682738380082,0.201847033339061));
#12842=CARTESIAN_POINT('Ctrl Pts',(11.6893150192885,1.40624834198077,0.403770984173611));
#12843=CARTESIAN_POINT('Ctrl Pts',(11.6791752715866,1.39566932719028,0.605694927437301));
#12844=CARTESIAN_POINT('',(11.6778970386953,1.39579479040469,0.605695249702977));
#12845=CARTESIAN_POINT('Ctrl Pts',(11.7095901160181,1.42740242188993,2.01986864734049E-16));
#12846=CARTESIAN_POINT('Ctrl Pts',(11.6990256725537,1.41686632615463,0.201898401304098));
#12847=CARTESIAN_POINT('Ctrl Pts',(11.6884613130147,1.40633044792991,0.403796817797553));
#12848=CARTESIAN_POINT('Ctrl Pts',(11.6778970386953,1.39579479040469,0.605695249702978));
#12849=CARTESIAN_POINT('Ctrl Pts',(11.6778970386953,1.39579479040469,0.605695249702977));
#12850=CARTESIAN_POINT('Ctrl Pts',(11.585279512325,1.40488700096013,0.605683574233495));
#12851=CARTESIAN_POINT('Ctrl Pts',(11.4926474653491,1.41386220753305,0.605671932550561));
#12852=CARTESIAN_POINT('Ctrl Pts',(11.4,1.4227102204299,0.605660349289938));
#12853=CARTESIAN_POINT('Origin',(7.9,1.7737037037037,0.));
#12854=CARTESIAN_POINT('',(7.9,-1.67543132363858,0.605300614462415));
#12855=CARTESIAN_POINT('Ctrl Pts',(7.9,-1.67543132363858,0.605300614462415));
#12856=CARTESIAN_POINT('Ctrl Pts',(7.9,-1.68078196203297,0.504592238472094));
#12857=CARTESIAN_POINT('Ctrl Pts',(7.9,-1.68613236521525,0.403883028813119));
#12858=CARTESIAN_POINT('Ctrl Pts',(7.9,-1.69685110017509,0.202116711316755));
#12859=CARTESIAN_POINT('Ctrl Pts',(7.9,-1.70221951791351,0.10105794916591));
#12860=CARTESIAN_POINT('Ctrl Pts',(7.9,-1.70758761671949,0.));
#12861=CARTESIAN_POINT('',(7.9,-1.57547905376932,0.7));
#12862=CARTESIAN_POINT('Ctrl Pts',(7.9,-1.57547905376882,0.7));
#12863=CARTESIAN_POINT('Ctrl Pts',(7.9,-1.58339333479856,0.700000000000001));
#12864=CARTESIAN_POINT('Ctrl Pts',(7.89999913038498,-1.59124411312484,0.699006032637452));
#12865=CARTESIAN_POINT('Ctrl Pts',(7.89999837104309,-1.59889106951376,0.697118831203047));
#12866=CARTESIAN_POINT('Ctrl Pts',(7.89999794343345,-1.6031973145812,0.696056087876834));
#12867=CARTESIAN_POINT('Ctrl Pts',(7.89999755365678,-1.60743898057435,0.694709047589066));
#12868=CARTESIAN_POINT('Ctrl Pts',(7.89999730661842,-1.61158931211603,0.693088720937666));
#12869=CARTESIAN_POINT('Ctrl Pts',(7.89999686465941,-1.6190143793929,0.690189908089508));
#12870=CARTESIAN_POINT('Ctrl Pts',(7.89999696143539,-1.626066934352,0.686450944759811));
#12871=CARTESIAN_POINT('Ctrl Pts',(7.89999752554231,-1.63260082031789,0.681953255064161));
#12872=CARTESIAN_POINT('Ctrl Pts',(7.89999783650325,-1.63620259020663,0.679473927540052));
#12873=CARTESIAN_POINT('Ctrl Pts',(7.89999827825103,-1.63964648551863,0.676763160200805));
#12874=CARTESIAN_POINT('Ctrl Pts',(7.89999867021687,-1.64290407802379,0.673829034208746));
#12875=CARTESIAN_POINT('Ctrl Pts',(7.89999905115172,-1.64606999298761,0.670977482527793));
#12876=CARTESIAN_POINT('Ctrl Pts',(7.89999938859403,-1.64904076201529,0.667932171841817));
#12877=CARTESIAN_POINT('Ctrl Pts',(7.89999938783828,-1.6517939440564,0.66470449824639));
#12878=CARTESIAN_POINT('Ctrl Pts',(7.89999938643498,-1.65690611124346,0.658711285012161));
#12879=CARTESIAN_POINT('Ctrl Pts',(7.89999834643869,-1.661271022418,0.652090721578155));
#12880=CARTESIAN_POINT('Ctrl Pts',(7.89999799057748,-1.66482884904143,0.645008203309728));
#12881=CARTESIAN_POINT('Ctrl Pts',(7.89999795399159,-1.66519462718329,0.644280053614395));
#12882=CARTESIAN_POINT('Ctrl Pts',(7.89999792287445,-1.66555183396469,0.643547001244109));
#12883=CARTESIAN_POINT('Ctrl Pts',(7.89999789784292,-1.66590037542058,0.642809214685104));
#12884=CARTESIAN_POINT('Ctrl Pts',(7.89999765441981,-1.66928982250308,0.635634491398386));
#12885=CARTESIAN_POINT('Ctrl Pts',(7.89999817709027,-1.67182454272713,0.628096763436417));
#12886=CARTESIAN_POINT('Ctrl Pts',(7.8999989464625,-1.67345106343068,0.620364350320046));
#12887=CARTESIAN_POINT('Ctrl Pts',(7.89999943944948,-1.67449328136075,0.615409688768565));
#12888=CARTESIAN_POINT('Ctrl Pts',(7.89999999630063,-1.67516175160204,0.610374426093907));
#12889=CARTESIAN_POINT('Ctrl Pts',(7.89999999769359,-1.67543132314592,0.605300614465834));
#12890=CARTESIAN_POINT('',(7.9,1.57547905376882,0.7));
#12891=CARTESIAN_POINT('',(7.9,0.886851851851852,0.7));
#12892=CARTESIAN_POINT('',(7.9,1.67543132363858,0.605300614462415));
#12893=CARTESIAN_POINT('Ctrl Pts',(7.89999999769359,1.67543132314592,0.605300614465834));
#12894=CARTESIAN_POINT('Ctrl Pts',(7.89999999552123,1.67501091691767,0.613213400729193));
#12895=CARTESIAN_POINT('Ctrl Pts',(7.89999875799714,1.67362284400845,0.621034919585595));
#12896=CARTESIAN_POINT('Ctrl Pts',(7.89999821041927,1.67135120200026,0.628604813990272));
#12897=CARTESIAN_POINT('Ctrl Pts',(7.89999790518813,1.67008494211401,0.632824428521627));
#12898=CARTESIAN_POINT('Ctrl Pts',(7.89999777089825,1.66854314417455,0.636965893954691));
#12899=CARTESIAN_POINT('Ctrl Pts',(7.89999784944871,1.66673368022774,0.640999456224326));
#12900=CARTESIAN_POINT('Ctrl Pts',(7.89999799035603,1.66348778281681,0.648235040746992));
#12901=CARTESIAN_POINT('Ctrl Pts',(7.8999989183875,1.65941887886545,0.655045206964536));
#12902=CARTESIAN_POINT('Ctrl Pts',(7.89999927807636,1.65459101651367,0.661266862646797));
#12903=CARTESIAN_POINT('Ctrl Pts',(7.89999934554656,1.65368540929837,0.662433916689859));
#12904=CARTESIAN_POINT('Ctrl Pts',(7.89999938740919,1.65275296801062,0.663580193269421));
#12905=CARTESIAN_POINT('Ctrl Pts',(7.89999938728957,1.65179394408007,0.664704498246374));
#12906=CARTESIAN_POINT('Ctrl Pts',(7.89999938705343,1.64990069294102,0.666924037937161));
#12907=CARTESIAN_POINT('Ctrl Pts',(7.89999922461202,1.64790387543569,0.669057997255949));
#12908=CARTESIAN_POINT('Ctrl Pts',(7.89999900301747,1.64581073954063,0.671102663899023));
#12909=CARTESIAN_POINT('Ctrl Pts',(7.89999840121276,1.64012621790684,0.676655553128015));
#12910=CARTESIAN_POINT('Ctrl Pts',(7.89999746538644,1.63379824275617,0.681490110487894));
#12911=CARTESIAN_POINT('Ctrl Pts',(7.89999715581736,1.6269906793715,0.685552192443336));
#12912=CARTESIAN_POINT('Ctrl Pts',(7.89999695885968,1.62265949106942,0.688136618155352));
#12913=CARTESIAN_POINT('Ctrl Pts',(7.89999697413705,1.61813320929371,0.690407672840119));
#12914=CARTESIAN_POINT('Ctrl Pts',(7.89999720528031,1.61344832872307,0.692342105328139));
#12915=CARTESIAN_POINT('Ctrl Pts',(7.89999756646959,1.60612763680413,0.69536488980882));
#12916=CARTESIAN_POINT('Ctrl Pts',(7.89999845750109,1.59850458633822,0.69753330980446));
#12917=CARTESIAN_POINT('Ctrl Pts',(7.89999917312139,1.59072625322659,0.698777780766876));
#12918=CARTESIAN_POINT('Ctrl Pts',(7.8999996358458,1.58569673594883,0.699582463224842));
#12919=CARTESIAN_POINT('Ctrl Pts',(7.9,1.58060170040825,0.7));
#12920=CARTESIAN_POINT('Ctrl Pts',(7.9,1.57547905376882,0.7));
#12921=CARTESIAN_POINT('Ctrl Pts',(7.9,1.70758761671949,0.));
#12922=CARTESIAN_POINT('Ctrl Pts',(7.9,1.70221949782947,0.101058327261027));
#12923=CARTESIAN_POINT('Ctrl Pts',(7.9,1.69685105999395,0.202117467714));
#12924=CARTESIAN_POINT('Ctrl Pts',(7.9,1.68613232500772,0.403883785628764));
#12925=CARTESIAN_POINT('Ctrl Pts',(7.9,1.6807819419292,0.504592616860323));
#12926=CARTESIAN_POINT('Ctrl Pts',(7.9,1.67543132363858,0.605300614462415));
#12927=CARTESIAN_POINT('Ctrl Pts',(7.91019312999368,-1.70715886092982,-0.000134090250286965));
#12928=CARTESIAN_POINT('Ctrl Pts',(7.90679525219671,-1.69658223918655,0.201692187253877));
#12929=CARTESIAN_POINT('Ctrl Pts',(7.90339729501941,-1.68600562260833,0.40351846369823));
#12930=CARTESIAN_POINT('Ctrl Pts',(7.89999925719352,-1.67542901130525,0.605344739067286));
#12931=CARTESIAN_POINT('Ctrl Pts',(6.63535348802246,-1.76179300886274,3.38453142643293E-5));
#12932=CARTESIAN_POINT('Ctrl Pts',(6.63422081661327,-1.7512156246026,0.201860399405878));
#12933=CARTESIAN_POINT('Ctrl Pts',(6.6330881724013,-1.74063821514668,0.403686949685767));
#12934=CARTESIAN_POINT('Ctrl Pts',(6.63195543348167,-1.7300608292057,0.605513504373875));
#12935=CARTESIAN_POINT('Ctrl Pts',(5.36191629096386,-1.76821426310706,6.25694230841134E-5));
#12936=CARTESIAN_POINT('Ctrl Pts',(5.36305144950513,-1.75763653444312,0.201889164820622));
#12937=CARTESIAN_POINT('Ctrl Pts',(5.36418670601529,-1.74705878452761,0.403715755186214));
#12938=CARTESIAN_POINT('Ctrl Pts',(5.36532191986746,-1.73648104871457,0.605542351516859));
#12939=CARTESIAN_POINT('Ctrl Pts',(4.08978435919194,-1.70060618495018,-0.000163379468877527));
#12940=CARTESIAN_POINT('Ctrl Pts',(4.09318947412453,-1.69002991101751,0.201662855819258));
#12941=CARTESIAN_POINT('Ctrl Pts',(4.09659468720556,-1.67945364498778,0.403489089874722));
#12942=CARTESIAN_POINT('Ctrl Pts',(4.1,-1.66887738702936,0.605315322680078));
#12943=CARTESIAN_POINT('Ctrl Pts',(4.10000000006189,-1.66887738587128,0.605315322687833));
#12944=CARTESIAN_POINT('Ctrl Pts',(5.36600428635239,-1.73653511802878,0.605201749988751));
#12945=CARTESIAN_POINT('Ctrl Pts',(6.63469107356441,-1.72995836404769,0.605216415547347));
#12946=CARTESIAN_POINT('Ctrl Pts',(7.89999999997453,-1.67543132304763,0.605300614465986));
#12947=CARTESIAN_POINT('Ctrl Pts',(7.9,-1.57547905376882,0.7));
#12948=CARTESIAN_POINT('Ctrl Pts',(6.63400208894818,-1.63014048526579,0.7));
#12949=CARTESIAN_POINT('Ctrl Pts',(5.36531976402288,-1.63670020240541,0.7));
#12950=CARTESIAN_POINT('Ctrl Pts',(4.09999999999999,-1.56887583540973,0.7));
#12951=CARTESIAN_POINT('Ctrl Pts',(7.9012470621039,-1.60436190544783,0.700000000000001));
#12952=CARTESIAN_POINT('Ctrl Pts',(6.6345175325877,-1.65907137725265,0.700000604190856));
#12953=CARTESIAN_POINT('Ctrl Pts',(5.36490325870521,-1.66564852467601,0.700000815814724));
#12954=CARTESIAN_POINT('Ctrl Pts',(4.09845273665223,-1.59774131518914,0.699999999999999));
#12955=CARTESIAN_POINT('Ctrl Pts',(7.90340849276168,-1.6544221878571,0.676636720659303));
#12956=CARTESIAN_POINT('Ctrl Pts',(6.63541917043928,-1.70921256696412,0.676609005714152));
#12957=CARTESIAN_POINT('Ctrl Pts',(5.36416860778507,-1.71581908642683,0.67660414986632));
#12958=CARTESIAN_POINT('Ctrl Pts',(4.09577098158984,-1.64777167791894,0.676641578059328));
#12959=CARTESIAN_POINT('Ctrl Pts',(7.90425799286387,-1.67409721877663,0.626952737571144));
#12960=CARTESIAN_POINT('Ctrl Pts',(6.63576820027036,-1.72888861107585,0.626881076846221));
#12961=CARTESIAN_POINT('Ctrl Pts',(5.36388821219926,-1.73550154452763,0.626868555890157));
#12962=CARTESIAN_POINT('Ctrl Pts',(4.09471668402893,-1.66744047248441,0.626965338598652));
#12963=CARTESIAN_POINT('Ctrl Pts',(7.90430757201307,-1.67524550738887,0.605300901379154));
#12964=CARTESIAN_POINT('Ctrl Pts',(6.63578978311492,-1.73002023206136,0.605216330280387));
#12965=CARTESIAN_POINT('Ctrl Pts',(5.3638700255334,-1.7366305488338,0.605201579557148));
#12966=CARTESIAN_POINT('Ctrl Pts',(4.09465499692593,-1.6685912965035,0.605315802949303));
#12967=CARTESIAN_POINT('Ctrl Pts',(7.9,-1.57547905376882,0.7));
#12968=CARTESIAN_POINT('Ctrl Pts',(6.63400208894818,-1.63014048526579,0.7));
#12969=CARTESIAN_POINT('Ctrl Pts',(5.36531976402288,-1.63670020240541,0.7));
#12970=CARTESIAN_POINT('Ctrl Pts',(4.09999999999999,-1.56887583540973,0.7));
#12971=CARTESIAN_POINT('Origin',(6.08012166120517,1.06778195214465E-16,
0.7));
#12972=CARTESIAN_POINT('Ctrl Pts',(4.1,1.56887583540973,0.7));
#12973=CARTESIAN_POINT('Ctrl Pts',(5.36531976402291,1.63670020240541,0.7));
#12974=CARTESIAN_POINT('Ctrl Pts',(6.63400208894819,1.63014048526579,0.7));
#12975=CARTESIAN_POINT('Ctrl Pts',(7.9,1.57547905376882,0.7));
#12976=CARTESIAN_POINT('Ctrl Pts',(4.1,1.56887583540973,0.7));
#12977=CARTESIAN_POINT('Ctrl Pts',(5.36531976402291,1.63670020240541,0.7));
#12978=CARTESIAN_POINT('Ctrl Pts',(6.63400208894819,1.63014048526579,0.7));
#12979=CARTESIAN_POINT('Ctrl Pts',(7.9,1.57547905376882,0.7));
#12980=CARTESIAN_POINT('Ctrl Pts',(4.09845273665224,1.59774131518914,0.699999999999999));
#12981=CARTESIAN_POINT('Ctrl Pts',(5.36490325870523,1.66564852467601,0.700000815814725));
#12982=CARTESIAN_POINT('Ctrl Pts',(6.6345175325877,1.65907137725265,0.700000604190856));
#12983=CARTESIAN_POINT('Ctrl Pts',(7.9012470621039,1.60436190544783,0.700000000000001));
#12984=CARTESIAN_POINT('Ctrl Pts',(4.09577098158985,1.64777167791894,0.676641578059328));
#12985=CARTESIAN_POINT('Ctrl Pts',(5.36416860778509,1.71581908642683,0.67660414986632));
#12986=CARTESIAN_POINT('Ctrl Pts',(6.6354191704393,1.70921256696412,0.676609005714152));
#12987=CARTESIAN_POINT('Ctrl Pts',(7.90340849276168,1.6544221878571,0.676636720659302));
#12988=CARTESIAN_POINT('Ctrl Pts',(4.09471668402895,1.66744047248441,0.626965338598652));
#12989=CARTESIAN_POINT('Ctrl Pts',(5.36388821219928,1.73550154452763,0.626868555890157));
#12990=CARTESIAN_POINT('Ctrl Pts',(6.63576820027036,1.72888861107585,0.626881076846221));
#12991=CARTESIAN_POINT('Ctrl Pts',(7.90425799286387,1.67409721877663,0.626952737571144));
#12992=CARTESIAN_POINT('Ctrl Pts',(4.09465499692594,1.6685912965035,0.605315802949303));
#12993=CARTESIAN_POINT('Ctrl Pts',(5.36387002553342,1.7366305488338,0.605201579557148));
#12994=CARTESIAN_POINT('Ctrl Pts',(6.63578978311492,1.73002023206136,0.605216330280387));
#12995=CARTESIAN_POINT('Ctrl Pts',(7.90430757201307,1.67524550738887,0.605300901379154));
#12996=CARTESIAN_POINT('Ctrl Pts',(7.89999999997454,1.67543132304763,0.605300614465986));
#12997=CARTESIAN_POINT('Ctrl Pts',(6.63469107356441,1.72995836404769,0.605216415547348));
#12998=CARTESIAN_POINT('Ctrl Pts',(5.36600428635241,1.73653511802878,0.605201749988751));
#12999=CARTESIAN_POINT('Ctrl Pts',(4.10000000006189,1.66887738587128,0.605315322687833));
#13000=CARTESIAN_POINT('Ctrl Pts',(4.08978435969213,1.70060618339657,-0.000163349821525811));
#13001=CARTESIAN_POINT('Ctrl Pts',(4.093189474458,1.69002990998177,0.201662875584159));
#13002=CARTESIAN_POINT('Ctrl Pts',(4.0965946873723,1.67945364446992,0.403489099757173));
#13003=CARTESIAN_POINT('Ctrl Pts',(4.1,1.66887738702936,0.605315322680078));
#13004=CARTESIAN_POINT('Ctrl Pts',(5.36191629113061,1.76821426155324,6.25990704884337E-5));
#13005=CARTESIAN_POINT('Ctrl Pts',(5.3630514496163,1.75763653340724,0.201889184585558));
#13006=CARTESIAN_POINT('Ctrl Pts',(5.36418670607087,1.74705878400967,0.403715765068683));
#13007=CARTESIAN_POINT('Ctrl Pts',(5.36532191986745,1.73648104871457,0.605542351516858));
#13008=CARTESIAN_POINT('Ctrl Pts',(6.63535348785608,1.76179300730897,3.38749616628245E-5));
#13009=CARTESIAN_POINT('Ctrl Pts',(6.63422081650235,1.75121562356675,0.20186041917081));
#13010=CARTESIAN_POINT('Ctrl Pts',(6.63308817234583,1.74063821462875,0.403686959568233));
#13011=CARTESIAN_POINT('Ctrl Pts',(6.63195543348166,1.7300608292057,0.605513504373875));
#13012=CARTESIAN_POINT('Ctrl Pts',(7.91019312949454,1.70715885937616,-0.000134060602928919));
#13013=CARTESIAN_POINT('Ctrl Pts',(7.90679525186394,1.69658223815078,0.201692207018782));
#13014=CARTESIAN_POINT('Ctrl Pts',(7.90339729485302,1.68600562209044,0.403518473580683));
#13015=CARTESIAN_POINT('Ctrl Pts',(7.89999925719352,1.67542901130525,0.605344739067286));
#13016=CARTESIAN_POINT('Origin',(3.9,1.7662962962963,0.));
#13017=CARTESIAN_POINT('',(3.9,-1.657567947596,0.605334330700044));
#13018=CARTESIAN_POINT('Ctrl Pts',(3.9,-1.657567947596,0.605334330700044));
#13019=CARTESIAN_POINT('Ctrl Pts',(3.9,-1.66295505583237,0.504667750148195));
#13020=CARTESIAN_POINT('Ctrl Pts',(3.9,-1.66834175427306,0.404000185805616));
#13021=CARTESIAN_POINT('Ctrl Pts',(3.9,-1.67913790341918,0.202222727053817));
#13022=CARTESIAN_POINT('Ctrl Pts',(3.9,-1.68454745406112,0.101110889248462));
#13023=CARTESIAN_POINT('Ctrl Pts',(3.9,-1.68995649764597,0.));
#13024=CARTESIAN_POINT('',(3.9,-1.55753217754889,0.7));
#13025=CARTESIAN_POINT('Ctrl Pts',(3.89999999700315,-1.55753217437,0.7));
#13026=CARTESIAN_POINT('Ctrl Pts',(3.89999999197785,-1.56545359401377,0.699999998841372));
#13027=CARTESIAN_POINT('Ctrl Pts',(3.90000117861029,-1.57331197233837,0.699006163267487));
#13028=CARTESIAN_POINT('Ctrl Pts',(3.90000221019459,-1.58096665047841,0.697118921400131));
#13029=CARTESIAN_POINT('Ctrl Pts',(3.90000279139136,-1.58527931230009,0.696055645348449));
#13030=CARTESIAN_POINT('Ctrl Pts',(3.90000331912093,-1.58952737074567,0.694707745526415));
#13031=CARTESIAN_POINT('Ctrl Pts',(3.90000364796674,-1.59368396010392,0.693086194530447));
#13032=CARTESIAN_POINT('Ctrl Pts',(3.90000423564848,-1.60111221870485,0.690188313817561));
#13033=CARTESIAN_POINT('Ctrl Pts',(3.90000407815102,-1.60816848972648,0.686450841450731));
#13034=CARTESIAN_POINT('Ctrl Pts',(3.9000032813392,-1.6147063365644,0.681954558458482));
#13035=CARTESIAN_POINT('Ctrl Pts',(3.90000284137901,-1.61831621321653,0.679471932695374));
#13036=CARTESIAN_POINT('Ctrl Pts',(3.90000222202081,-1.62176776859012,0.67675708350434));
#13037=CARTESIAN_POINT('Ctrl Pts',(3.9000016760669,-1.6250323621476,0.673818036286869));
#13038=CARTESIAN_POINT('Ctrl Pts',(3.90000114791654,-1.62819049732732,0.670974831382826));
#13039=CARTESIAN_POINT('Ctrl Pts',(3.90000068451114,-1.63115458712464,0.667938911589952));
#13040=CARTESIAN_POINT('Ctrl Pts',(3.90000068976928,-1.6339023205034,0.664721489040691));
#13041=CARTESIAN_POINT('Ctrl Pts',(3.90000069956116,-1.63901923218135,0.658729908073458));
#13042=CARTESIAN_POINT('Ctrl Pts',(3.9000021571807,-1.64338878348726,0.652110283780478));
#13043=CARTESIAN_POINT('Ctrl Pts',(3.90000267296827,-1.64695081636755,0.645027851744832));
#13044=CARTESIAN_POINT('Ctrl Pts',(3.90000272641596,-1.64731992654249,0.644293945625623));
#13045=CARTESIAN_POINT('Ctrl Pts',(3.90000277224081,-1.64768032438231,0.643555049900053));
#13046=CARTESIAN_POINT('Ctrl Pts',(3.90000280957334,-1.64803191324525,0.642811337026806));
#13047=CARTESIAN_POINT('Ctrl Pts',(3.90000316967295,-1.65142324611312,0.635637680016741));
#13048=CARTESIAN_POINT('Ctrl Pts',(3.90000247513984,-1.65395957542788,0.628100801230905));
#13049=CARTESIAN_POINT('Ctrl Pts',(3.90000142932204,-1.65558732484325,0.62036898832433));
#13050=CARTESIAN_POINT('Ctrl Pts',(3.90000076044003,-1.65662839749185,0.615423891207338));
#13051=CARTESIAN_POINT('Ctrl Pts',(3.9,-1.65729694754734,0.61039839235075));
#13052=CARTESIAN_POINT('Ctrl Pts',(3.9,-1.657567947596,0.605334330700044));
#13053=CARTESIAN_POINT('',(3.9,1.55753217754922,0.7));
#13054=CARTESIAN_POINT('',(3.9,0.883148148148148,0.7));
#13055=CARTESIAN_POINT('',(3.9,1.657567947596,0.605334330700044));
#13056=CARTESIAN_POINT('Ctrl Pts',(3.9,1.657567947596,0.605334330700044));
#13057=CARTESIAN_POINT('Ctrl Pts',(3.9,1.65714453107083,0.613246533660879));
#13058=CARTESIAN_POINT('Ctrl Pts',(3.90000169450566,1.65575314729854,0.621067109624563));
#13059=CARTESIAN_POINT('Ctrl Pts',(3.900002426785,1.653477907766,0.628635640467799));
#13060=CARTESIAN_POINT('Ctrl Pts',(3.90000283370343,1.65221358571927,0.632841378048222));
#13061=CARTESIAN_POINT('Ctrl Pts',(3.90000300372053,1.65067534627202,0.636969322077829));
#13062=CARTESIAN_POINT('Ctrl Pts',(3.90000288278183,1.6488710006323,0.640990000951852));
#13063=CARTESIAN_POINT('Ctrl Pts',(3.90000266510116,1.6456233127241,0.64822692378658));
#13064=CARTESIAN_POINT('Ctrl Pts',(3.90000136145047,1.64155197609259,0.655037842274187));
#13065=CARTESIAN_POINT('Ctrl Pts',(3.9000008487987,1.63672139510901,0.661259788874982));
#13066=CARTESIAN_POINT('Ctrl Pts',(3.90000075195303,1.63580884415802,0.662435184403355));
#13067=CARTESIAN_POINT('Ctrl Pts',(3.90000069125178,1.63486906637168,0.663589490553999));
#13068=CARTESIAN_POINT('Ctrl Pts',(3.90000068992127,1.63390232051248,0.664721489040685));
#13069=CARTESIAN_POINT('Ctrl Pts',(3.90000068733544,1.63202347103487,0.666921503393101));
#13070=CARTESIAN_POINT('Ctrl Pts',(3.9000009071255,1.6300427915863,0.669037305429552));
#13071=CARTESIAN_POINT('Ctrl Pts',(3.90000121037842,1.62796736695056,0.671065303566633));
#13072=CARTESIAN_POINT('Ctrl Pts',(3.90000204102081,1.62228255539437,0.676620208836154));
#13073=CARTESIAN_POINT('Ctrl Pts',(3.90000335328325,1.61595386407616,0.681456575151491));
#13074=CARTESIAN_POINT('Ctrl Pts',(3.90000380482706,1.60914557515952,0.685520902406533));
#13075=CARTESIAN_POINT('Ctrl Pts',(3.90000409284089,1.60480295930069,0.688113302965514));
#13076=CARTESIAN_POINT('Ctrl Pts',(3.90000408819389,1.6002642541482,0.690390927291682));
#13077=CARTESIAN_POINT('Ctrl Pts',(3.90000378365133,1.59556629223371,0.692330537597694));
#13078=CARTESIAN_POINT('Ctrl Pts',(3.90000330864444,1.58823869807682,0.695355823328757));
#13079=CARTESIAN_POINT('Ctrl Pts',(3.90000209726118,1.58060840086481,0.697526456028474));
#13080=CARTESIAN_POINT('Ctrl Pts',(3.90000112250675,1.5728228815436,0.698773197673241));
#13081=CARTESIAN_POINT('Ctrl Pts',(3.90000049100668,1.56777898966077,0.699580906164169));
#13082=CARTESIAN_POINT('Ctrl Pts',(3.89999999374416,1.56266934880282,0.69999999924861));
#13083=CARTESIAN_POINT('Ctrl Pts',(3.89999999700315,1.55753217437,0.7));
#13084=CARTESIAN_POINT('Ctrl Pts',(3.9,1.68995649764597,0.));
#13085=CARTESIAN_POINT('Ctrl Pts',(3.9,1.68454744095908,0.101111134163871));
#13086=CARTESIAN_POINT('Ctrl Pts',(3.9,1.67913787721413,0.202223216861756));
#13087=CARTESIAN_POINT('Ctrl Pts',(3.9,1.66834172806373,0.404000675610066));
#13088=CARTESIAN_POINT('Ctrl Pts',(3.9,1.66295504272671,0.504667995047933));
#13089=CARTESIAN_POINT('Ctrl Pts',(3.9,1.657567947596,0.605334330700044));
#13090=CARTESIAN_POINT('Ctrl Pts',(3.90000000000029,-1.68995649764598,2.25514051876985E-17));
#13091=CARTESIAN_POINT('Ctrl Pts',(3.90375240214247,-1.67935614215062,0.202290156525516));
#13092=CARTESIAN_POINT('Ctrl Pts',(3.90750491350916,-1.66875579641967,0.404580311547879));
#13093=CARTESIAN_POINT('Ctrl Pts',(3.91125753584366,-1.65815546066147,0.606870465045848));
#13094=CARTESIAN_POINT('Ctrl Pts',(2.95719731373254,-1.63434162994996,-0.000186284957671625));
#13095=CARTESIAN_POINT('Ctrl Pts',(2.96263618266967,-1.62374249289717,0.202103577800055));
#13096=CARTESIAN_POINT('Ctrl Pts',(2.96807524459186,-1.6131433886527,0.404393433349269));
#13097=CARTESIAN_POINT('Ctrl Pts',(2.97351444051957,-1.60254429060724,0.606683290324339));
#13098=CARTESIAN_POINT('Ctrl Pts',(2.0151035222252,-1.5373601393942,-0.000515615972119944));
#13099=CARTESIAN_POINT('Ctrl Pts',(2.0222299762717,-1.52676329064944,0.20177372753372));
#13100=CARTESIAN_POINT('Ctrl Pts',(2.02935668076532,-1.51616649670304,0.404063061036967));
#13101=CARTESIAN_POINT('Ctrl Pts',(2.03648357820815,-1.50556972342972,0.606352393906678));
#13102=CARTESIAN_POINT('Ctrl Pts',(1.07355614839761,-1.3885225322474,-0.00102014041634142));
#13103=CARTESIAN_POINT('Ctrl Pts',(1.08237048982668,-1.37792954541675,0.201268457136957));
#13104=CARTESIAN_POINT('Ctrl Pts',(1.09118510562603,-1.36733662501784,0.403557046289628));
#13105=CARTESIAN_POINT('Ctrl Pts',(1.09999999998551,-1.35674377243019,0.605845626932519));
#13106=CARTESIAN_POINT('Ctrl Pts',(1.10000000359112,-1.35674374984279,0.605845627045242));
#13107=CARTESIAN_POINT('Ctrl Pts',(2.02777573897866,-1.50422778688462,0.60559460123127));
#13108=CARTESIAN_POINT('Ctrl Pts',(2.96295221054883,-1.60165319397541,0.605428415101273));
#13109=CARTESIAN_POINT('Ctrl Pts',(3.9,-1.657567947596,0.605334330700044));
#13110=CARTESIAN_POINT('Ctrl Pts',(3.90594750914669,-1.55788759822396,0.7));
#13111=CARTESIAN_POINT('Ctrl Pts',(2.96654482017732,-1.50183737247472,0.7));
#13112=CARTESIAN_POINT('Ctrl Pts',(2.02939151553635,-1.40396309164617,0.7));
#13113=CARTESIAN_POINT('Ctrl Pts',(1.1,-1.25565664448621,0.7));
#13114=CARTESIAN_POINT('Ctrl Pts',(3.90422602671531,-1.58673967158186,0.7));
#13115=CARTESIAN_POINT('Ctrl Pts',(2.9639697519154,-1.53062009474021,0.699999324449154));
#13116=CARTESIAN_POINT('Ctrl Pts',(2.02587169016863,-1.43262076012027,0.700001792708215));
#13117=CARTESIAN_POINT('Ctrl Pts',(1.09546090287069,-1.28410178925883,0.700000000000001));
#13118=CARTESIAN_POINT('Ctrl Pts',(3.90124198563808,-1.6367522482393,0.676652244116846));
#13119=CARTESIAN_POINT('Ctrl Pts',(2.95951584878018,-1.58051528054544,0.676683243227538));
#13120=CARTESIAN_POINT('Ctrl Pts',(2.01975879699698,-1.48229505764113,0.676737195552829));
#13121=CARTESIAN_POINT('Ctrl Pts',(1.08759175402576,-1.33341535796084,0.676819902351873));
#13122=CARTESIAN_POINT('Ctrl Pts',(3.90006887217438,-1.65641364884095,0.626981005337021));
#13123=CARTESIAN_POINT('Ctrl Pts',(2.95775794493813,-1.6001648299169,0.627061170854983));
#13124=CARTESIAN_POINT('Ctrl Pts',(2.01735267249256,-1.50192280897576,0.627202240820629));
#13125=CARTESIAN_POINT('Ctrl Pts',(1.08446813262788,-1.35299014570964,0.627416665943555));
#13126=CARTESIAN_POINT('Ctrl Pts',(3.9,-1.657567947596,0.605334330700044));
#13127=CARTESIAN_POINT('Ctrl Pts',(2.95765589353472,-1.60133715645388,0.605428946878649));
#13128=CARTESIAN_POINT('Ctrl Pts',(2.01720431860088,-1.50312513840151,0.605596482146283));
#13129=CARTESIAN_POINT('Ctrl Pts',(1.0842689834292,-1.35423815332579,0.605849891671036));
#13130=CARTESIAN_POINT('Ctrl Pts',(3.89999999700313,-1.55753217437,0.7));
#13131=CARTESIAN_POINT('Ctrl Pts',(2.96258932077475,-1.50142404037792,0.7));
#13132=CARTESIAN_POINT('Ctrl Pts',(2.02743012901897,-1.40365010593343,0.7));
#13133=CARTESIAN_POINT('Ctrl Pts',(1.1,-1.25565664448621,0.7));
#13134=CARTESIAN_POINT('Origin',(6.08012166120517,1.06778195214465E-16,
0.7));
#13135=CARTESIAN_POINT('Ctrl Pts',(1.1,1.25565664448621,0.7));
#13136=CARTESIAN_POINT('Ctrl Pts',(2.02743012901899,1.40365010593344,0.7));
#13137=CARTESIAN_POINT('Ctrl Pts',(2.96258932077472,1.50142404037792,0.7));
#13138=CARTESIAN_POINT('Ctrl Pts',(3.89999999700315,1.55753217437,0.7));
#13139=CARTESIAN_POINT('Ctrl Pts',(1.1,1.25565664448621,0.7));
#13140=CARTESIAN_POINT('Ctrl Pts',(2.02939151553637,1.40396309164617,0.7));
#13141=CARTESIAN_POINT('Ctrl Pts',(2.96654482017727,1.50183737247472,0.7));
#13142=CARTESIAN_POINT('Ctrl Pts',(3.90594750914669,1.55788759822396,0.7));
#13143=CARTESIAN_POINT('Ctrl Pts',(1.09546090287069,1.28410178925883,0.700000000000001));
#13144=CARTESIAN_POINT('Ctrl Pts',(2.02587169016866,1.43262076012027,0.700001792708215));
#13145=CARTESIAN_POINT('Ctrl Pts',(2.96396975191535,1.53062009474021,0.699999324449154));
#13146=CARTESIAN_POINT('Ctrl Pts',(3.90422602671531,1.58673967158186,0.7));
#13147=CARTESIAN_POINT('Ctrl Pts',(1.08759175402576,1.33341535796084,0.676819902351873));
#13148=CARTESIAN_POINT('Ctrl Pts',(2.019758796997,1.48229505764113,0.676737195552829));
#13149=CARTESIAN_POINT('Ctrl Pts',(2.95951584878014,1.58051528054544,0.676683243227538));
#13150=CARTESIAN_POINT('Ctrl Pts',(3.90124198563808,1.6367522482393,0.676652244116846));
#13151=CARTESIAN_POINT('Ctrl Pts',(1.08446813262788,1.35299014570964,0.627416665943555));
#13152=CARTESIAN_POINT('Ctrl Pts',(2.01735267249258,1.50192280897576,0.627202240820629));
#13153=CARTESIAN_POINT('Ctrl Pts',(2.95775794493809,1.6001648299169,0.627061170854983));
#13154=CARTESIAN_POINT('Ctrl Pts',(3.90006887217438,1.65641364884095,0.626981005337021));
#13155=CARTESIAN_POINT('Ctrl Pts',(1.0842689834292,1.35423815332579,0.605849891671036));
#13156=CARTESIAN_POINT('Ctrl Pts',(2.0172043186009,1.50312513840152,0.605596482146283));
#13157=CARTESIAN_POINT('Ctrl Pts',(2.95765589353468,1.60133715645387,0.605428946878649));
#13158=CARTESIAN_POINT('Ctrl Pts',(3.9,1.657567947596,0.605334330700044));
#13159=CARTESIAN_POINT('Ctrl Pts',(3.9,1.657567947596,0.605334330700044));
#13160=CARTESIAN_POINT('Ctrl Pts',(2.96295221054879,1.60165319397541,0.605428415101273));
#13161=CARTESIAN_POINT('Ctrl Pts',(2.02777573897867,1.50422778688462,0.60559460123127));
#13162=CARTESIAN_POINT('Ctrl Pts',(1.10000000359111,1.35674374984279,0.605845627045242));
#13163=CARTESIAN_POINT('Ctrl Pts',(1.07355614839761,1.3885225322474,-0.00102014041634139));
#13164=CARTESIAN_POINT('Ctrl Pts',(1.08237048982668,1.37792954541676,0.201268457136957));
#13165=CARTESIAN_POINT('Ctrl Pts',(1.09118510562602,1.36733662501784,0.403557046289628));
#13166=CARTESIAN_POINT('Ctrl Pts',(1.09999999998551,1.35674377243019,0.605845626932519));
#13167=CARTESIAN_POINT('Ctrl Pts',(2.0151035222252,1.5373601393942,-0.000515615972119942));
#13168=CARTESIAN_POINT('Ctrl Pts',(2.0222299762717,1.52676329064944,0.201773727533721));
#13169=CARTESIAN_POINT('Ctrl Pts',(2.02935668076532,1.51616649670304,0.404063061036968));
#13170=CARTESIAN_POINT('Ctrl Pts',(2.03648357820815,1.50556972342972,0.606352393906678));
#13171=CARTESIAN_POINT('Ctrl Pts',(2.95719731373254,1.63434162994996,-0.000186284957671606));
#13172=CARTESIAN_POINT('Ctrl Pts',(2.96263618266967,1.62374249289717,0.202103577800055));
#13173=CARTESIAN_POINT('Ctrl Pts',(2.96807524459186,1.6131433886527,0.404393433349269));
#13174=CARTESIAN_POINT('Ctrl Pts',(2.97351444051957,1.60254429060724,0.60668329032434));
#13175=CARTESIAN_POINT('Ctrl Pts',(3.90000000000029,1.68995649764598,4.33680868994202E-17));
#13176=CARTESIAN_POINT('Ctrl Pts',(3.90375240214247,1.67935614215062,0.202290156525516));
#13177=CARTESIAN_POINT('Ctrl Pts',(3.90750491350917,1.66875579641967,0.404580311547879));
#13178=CARTESIAN_POINT('Ctrl Pts',(3.91125753584366,1.65815546066147,0.606870465045848));
#13179=CARTESIAN_POINT('Origin',(0.9,1.44962962962963,0.));
#13180=CARTESIAN_POINT('',(0.900000000000025,-1.32415632515176,0.605901073595307));
#13181=CARTESIAN_POINT('Ctrl Pts',(0.900000000000025,-1.32415632515176,
0.605901073595307));
#13182=CARTESIAN_POINT('Ctrl Pts',(0.900000000000025,-1.33021622058432,
0.504787384877132));
#13183=CARTESIAN_POINT('Ctrl Pts',(0.900000000000001,-1.33627289299046,
0.403672458220672));
#13184=CARTESIAN_POINT('Ctrl Pts',(0.900000000000001,-1.3483639425303,0.201706128802639));
#13185=CARTESIAN_POINT('Ctrl Pts',(0.9,-1.3543984610184,0.100852646477479));
#13186=CARTESIAN_POINT('Ctrl Pts',(0.9,-1.3604297237941,0.));
#13187=CARTESIAN_POINT('',(0.9,-1.22294421121193,0.7));
#13188=CARTESIAN_POINT('Ctrl Pts',(0.899999998934589,-1.2229442093848,0.7));
#13189=CARTESIAN_POINT('Ctrl Pts',(0.89999998269596,-1.2309559991361,0.699999991698178));
#13190=CARTESIAN_POINT('Ctrl Pts',(0.900003161357076,-1.2389110096839,0.699008412490225));
#13191=CARTESIAN_POINT('Ctrl Pts',(0.900005837532895,-1.24666554379878,
0.697120920272419));
#13192=CARTESIAN_POINT('Ctrl Pts',(0.900007138246235,-1.25043451364619,
0.69620353424371));
#13193=CARTESIAN_POINT('Ctrl Pts',(0.900008321383585,-1.25415610217771,
0.695073675615989));
#13194=CARTESIAN_POINT('Ctrl Pts',(0.900009136546862,-1.25781268161099,
0.69373809091454));
#13195=CARTESIAN_POINT('Ctrl Pts',(0.90001081442992,-1.26533916477404,0.690989003700189));
#13196=CARTESIAN_POINT('Ctrl Pts',(0.900010659344479,-1.27251458345821,
0.687399440976464));
#13197=CARTESIAN_POINT('Ctrl Pts',(0.900008585023094,-1.27919110928202,
0.68304500924512));
#13198=CARTESIAN_POINT('Ctrl Pts',(0.900007251085311,-1.28348459539356,
0.680244796581297));
#13199=CARTESIAN_POINT('Ctrl Pts',(0.900005156998288,-1.28757155292352,
0.67712723751572));
#13200=CARTESIAN_POINT('Ctrl Pts',(0.900003422242992,-1.29140570811059,
0.673703384872626));
#13201=CARTESIAN_POINT('Ctrl Pts',(0.90000203719427,-1.29446694202502,0.670969741262059));
#13202=CARTESIAN_POINT('Ctrl Pts',(0.90000088611098,-1.29734878548314,0.668056850549005));
#13203=CARTESIAN_POINT('Ctrl Pts',(0.900000936626746,-1.30003070819003,
0.664973821719563));
#13204=CARTESIAN_POINT('Ctrl Pts',(0.90000103432908,-1.30521780373233,0.659010948495488));
#13205=CARTESIAN_POINT('Ctrl Pts',(0.900005119671874,-1.30966005175478,
0.652412896960716));
#13206=CARTESIAN_POINT('Ctrl Pts',(0.900006662646281,-1.31329014967729,
0.64534035177384));
#13207=CARTESIAN_POINT('Ctrl Pts',(0.900006837929091,-1.31370253096037,
0.644536906434065));
#13208=CARTESIAN_POINT('Ctrl Pts',(0.900006988901759,-1.3141043809937,0.64372731654354));
#13209=CARTESIAN_POINT('Ctrl Pts',(0.900007112770807,-1.31449556093743,
0.642911804846506));
#13210=CARTESIAN_POINT('Ctrl Pts',(0.900008198175579,-1.31792328224658,
0.635765868899185));
#13211=CARTESIAN_POINT('Ctrl Pts',(0.900006415208278,-1.32049402672979,
0.628253543462219));
#13212=CARTESIAN_POINT('Ctrl Pts',(0.900003664797616,-1.32215034643222,
0.620540220943237));
#13213=CARTESIAN_POINT('Ctrl Pts',(0.900001948338234,-1.32318401225236,
0.615726538031782));
#13214=CARTESIAN_POINT('Ctrl Pts',(0.900000000000001,-1.32386068836271,
0.610833984830158));
#13215=CARTESIAN_POINT('Ctrl Pts',(0.900000000000001,-1.32415632515176,
0.605901073595307));
#13216=CARTESIAN_POINT('',(0.9,1.22294421121193,0.7));
#13217=CARTESIAN_POINT('',(0.9,0.724814814814815,0.7));
#13218=CARTESIAN_POINT('',(0.900000000000027,1.32415632515176,0.605901073595307));
#13219=CARTESIAN_POINT('Ctrl Pts',(0.900000000000001,1.32415632515176,0.605901073595307));
#13220=CARTESIAN_POINT('Ctrl Pts',(0.900000000000001,1.32368299187747,0.613798977756921));
#13221=CARTESIAN_POINT('Ctrl Pts',(0.900004523569871,1.32223544152535,0.621596324701597));
#13222=CARTESIAN_POINT('Ctrl Pts',(0.900006356724635,1.31990036466821,0.629134362570908));
#13223=CARTESIAN_POINT('Ctrl Pts',(0.900007328861843,1.3186620540024,0.633131846706937));
#13224=CARTESIAN_POINT('Ctrl Pts',(0.900007702029268,1.31717322147439,0.637056437951431));
#13225=CARTESIAN_POINT('Ctrl Pts',(0.900007358328755,1.31544117393516,0.640882963165587));
#13226=CARTESIAN_POINT('Ctrl Pts',(0.900006707239278,1.31216006761937,0.648131745755711));
#13227=CARTESIAN_POINT('Ctrl Pts',(0.900003091243194,1.3080468004769,0.654946293188228));
#13228=CARTESIAN_POINT('Ctrl Pts',(0.900001489347898,1.30317324258861,0.661167512355852));
#13229=CARTESIAN_POINT('Ctrl Pts',(0.900001155878064,1.30215870403359,0.662462596327245));
#13230=CARTESIAN_POINT('Ctrl Pts',(0.90000093695446,1.30111105636563,0.663731893727214));
#13231=CARTESIAN_POINT('Ctrl Pts',(0.90000091848414,1.30003070515708,0.664973821721807));
#13232=CARTESIAN_POINT('Ctrl Pts',(0.90000089007412,1.29836896897911,0.666884086330845));
#13233=CARTESIAN_POINT('Ctrl Pts',(0.900001333486324,1.29662987445651,0.668729618924651));
#13234=CARTESIAN_POINT('Ctrl Pts',(0.900001997973453,1.2948182721625,0.670508241825176));
#13235=CARTESIAN_POINT('Ctrl Pts',(0.900004083621534,1.28913213515815,0.676090865298813));
#13236=CARTESIAN_POINT('Ctrl Pts',(0.900007925915178,1.28279871831387,0.680954424681199));
#13237=CARTESIAN_POINT('Ctrl Pts',(0.900009431597099,1.27598654051802,0.685053039288488));
#13238=CARTESIAN_POINT('Ctrl Pts',(0.900010426918848,1.2714833923965,0.687762403198649));
#13239=CARTESIAN_POINT('Ctrl Pts',(0.900010579450444,1.26676996242859,0.690136867340003));
#13240=CARTESIAN_POINT('Ctrl Pts',(0.900009885932263,1.26188774903006,0.692153145632694));
#13241=CARTESIAN_POINT('Ctrl Pts',(0.900008832351734,1.25447077696631,0.695216239878874));
#13242=CARTESIAN_POINT('Ctrl Pts',(0.900005746465811,1.24674633448708,0.697421320974322));
#13243=CARTESIAN_POINT('Ctrl Pts',(0.900003140090462,1.23886595492982,0.6987028844583));
#13244=CARTESIAN_POINT('Ctrl Pts',(0.900001403206082,1.23361448254879,0.699556916322089));
#13245=CARTESIAN_POINT('Ctrl Pts',(0.899999988093253,1.22829309040712,0.699999994457486));
#13246=CARTESIAN_POINT('Ctrl Pts',(0.899999998934588,1.2229442093848,0.7));
#13247=CARTESIAN_POINT('Ctrl Pts',(0.9,1.3604297237941,0.));
#13248=CARTESIAN_POINT('Ctrl Pts',(0.9,1.35439838926384,0.100853846331769));
#13249=CARTESIAN_POINT('Ctrl Pts',(0.9,1.34836379894337,0.201708528537181));
#13250=CARTESIAN_POINT('Ctrl Pts',(0.9,1.33627274925098,0.403674857922336));
#13251=CARTESIAN_POINT('Ctrl Pts',(0.900000000000027,1.33021614867672,0.504788584706939));
#13252=CARTESIAN_POINT('Ctrl Pts',(0.900000000000027,1.32415632515176,0.605901073595307));
#13253=CARTESIAN_POINT('Ctrl Pts',(0.900000000000001,-1.3604297237941,-1.73472347597681E-18));
#13254=CARTESIAN_POINT('Ctrl Pts',(0.909119345746934,-1.34984469470005,
0.202150401646216));
#13255=CARTESIAN_POINT('Ctrl Pts',(0.918238975454288,-1.33925973741039,
0.404300794324169));
#13256=CARTESIAN_POINT('Ctrl Pts',(0.92735889343571,-1.32867485341111,0.606451177918334));
#13257=CARTESIAN_POINT('Ctrl Pts',(0.693791632045388,-1.32642527651154,
-0.000115194085079675));
#13258=CARTESIAN_POINT('Ctrl Pts',(0.703280422539661,-1.31584113310577,
0.202035038813999));
#13259=CARTESIAN_POINT('Ctrl Pts',(0.712769508818954,-1.30525706820637,
0.404185262036053));
#13260=CARTESIAN_POINT('Ctrl Pts',(0.722258895242942,-1.29467308328318,
0.606335475483814));
#13261=CARTESIAN_POINT('Ctrl Pts',(0.487608314405001,-1.28990207050556,
-0.000238777108575344));
#13262=CARTESIAN_POINT('Ctrl Pts',(0.497466558273561,-1.27931888757273,
0.201911276725417));
#13263=CARTESIAN_POINT('Ctrl Pts',(0.507325109482935,-1.26873579028159,
0.404061320158324));
#13264=CARTESIAN_POINT('Ctrl Pts',(0.517183972542757,-1.25815278023897,
0.606211353085106));
#13265=CARTESIAN_POINT('Ctrl Pts',(0.281447431601629,-1.2507496025167,-0.000370926150909055));
#13266=CARTESIAN_POINT('Ctrl Pts',(0.291675125201343,-1.24016745708839,
0.201778938960696));
#13267=CARTESIAN_POINT('Ctrl Pts',(0.301903137322998,-1.2295854048496,0.403928792940867));
#13268=CARTESIAN_POINT('Ctrl Pts',(0.312131472716966,-1.21900344770756,
0.606078635650713));
#13269=CARTESIAN_POINT('',(0.313137632044026,-1.21919552599285,0.606079286803921));
#13270=CARTESIAN_POINT('Ctrl Pts',(0.28146619846596,-1.25073018526678,-6.36968776335234E-17));
#13271=CARTESIAN_POINT('Ctrl Pts',(0.292023490345879,-1.2402182973453,0.20202640462578));
#13272=CARTESIAN_POINT('Ctrl Pts',(0.302580635585432,-1.22970674279184,
0.404052833452346));
#13273=CARTESIAN_POINT('Ctrl Pts',(0.313137632044028,-1.21919552599286,
0.606079286803922));
#13274=CARTESIAN_POINT('Ctrl Pts',(0.313137632044026,-1.21919552599285,
0.606079286803921));
#13275=CARTESIAN_POINT('Ctrl Pts',(0.508347756773358,-1.25646926692181,
0.606016122348466));
#13276=CARTESIAN_POINT('Ctrl Pts',(0.703992099548353,-1.29143758865737,
0.605956720831638));
#13277=CARTESIAN_POINT('Ctrl Pts',(0.900000000000031,-1.32415632515176,
0.605901073595307));
#13278=CARTESIAN_POINT('Ctrl Pts',(0.916434425702686,-1.22569269236154,
0.7));
#13279=CARTESIAN_POINT('Ctrl Pts',(0.72117838049967,-1.193102781986,0.7));
#13280=CARTESIAN_POINT('Ctrl Pts',(0.526295996270969,-1.15827411715321,
0.7));
#13281=CARTESIAN_POINT('Ctrl Pts',(0.3318563713692,-1.12115139781564,0.7));
#13282=CARTESIAN_POINT('Ctrl Pts',(0.911693828447622,-1.25409504944868,
0.700000000000001));
#13283=CARTESIAN_POINT('Ctrl Pts',(0.716221724293519,-1.22145811194286,
0.699999606692487));
#13284=CARTESIAN_POINT('Ctrl Pts',(0.52112301919326,-1.18657973614434,0.700000445015345));
#13285=CARTESIAN_POINT('Ctrl Pts',(0.32646265058614,-1.14940237362229,0.699999999999999));
#13286=CARTESIAN_POINT('Ctrl Pts',(0.903473253113197,-1.30334701150065,
0.676847307332805));
#13287=CARTESIAN_POINT('Ctrl Pts',(0.707628846166824,-1.27063023858114,
0.676865462359186));
#13288=CARTESIAN_POINT('Ctrl Pts',(0.512149925983835,-1.23566412474798,
0.676884474751893));
#13289=CARTESIAN_POINT('Ctrl Pts',(0.317109102097966,-1.19839394783867,
0.676905055067496));
#13290=CARTESIAN_POINT('Ctrl Pts',(0.900209809599689,-1.32289929215588,
0.627459885485154));
#13291=CARTESIAN_POINT('Ctrl Pts',(0.704212910592823,-1.29017057588713,
0.627506965865002));
#13292=CARTESIAN_POINT('Ctrl Pts',(0.50858160780484,-1.25519230329596,0.627556915196293));
#13293=CARTESIAN_POINT('Ctrl Pts',(0.31338355686088,-1.21790743260971,0.627610331402299));
#13294=CARTESIAN_POINT('Ctrl Pts',(0.900000000000031,-1.32415632515176,
0.605901073595307));
#13295=CARTESIAN_POINT('Ctrl Pts',(0.703992099548353,-1.29143758865737,
0.605956720831638));
#13296=CARTESIAN_POINT('Ctrl Pts',(0.508347756773358,-1.25646926692181,
0.606016122348466));
#13297=CARTESIAN_POINT('Ctrl Pts',(0.313137632044026,-1.21919552599285,
0.606079286803921));
#13298=CARTESIAN_POINT('',(0.3318563713692,-1.12115139781563,0.7));
#13299=CARTESIAN_POINT('Origin',(0.331856371369202,-1.12115139781563,0.6));
#13300=CARTESIAN_POINT('Ctrl Pts',(0.899999998934586,-1.2229442093848,0.7));
#13301=CARTESIAN_POINT('Ctrl Pts',(0.71024282334811,-1.19114655107378,0.7));
#13302=CARTESIAN_POINT('Ctrl Pts',(0.520840466228891,-1.15723253876768,
0.7));
#13303=CARTESIAN_POINT('Ctrl Pts',(0.3318563713692,-1.12115139781564,0.7));
#13304=CARTESIAN_POINT('Origin',(6.08012166120517,1.06778195214465E-16,
0.7));
#13305=CARTESIAN_POINT('',(0.331856371369203,1.12115139781563,0.7));
#13306=CARTESIAN_POINT('',(0.3318563713692,-0.7,0.7));
#13307=CARTESIAN_POINT('Ctrl Pts',(0.331856371369202,1.12115139781564,0.7));
#13308=CARTESIAN_POINT('Ctrl Pts',(0.520840466228894,1.15723253876768,0.7));
#13309=CARTESIAN_POINT('Ctrl Pts',(0.710242823348114,1.19114655107378,0.7));
#13310=CARTESIAN_POINT('Ctrl Pts',(0.899999998934589,1.2229442093848,0.7));
#13311=CARTESIAN_POINT('Ctrl Pts',(0.281447431601628,1.2507496025167,-0.000370926150909064));
#13312=CARTESIAN_POINT('Ctrl Pts',(0.291675125201342,1.24016745708839,0.201778938960695));
#13313=CARTESIAN_POINT('Ctrl Pts',(0.301903137322998,1.2295854048496,0.403928792940867));
#13314=CARTESIAN_POINT('Ctrl Pts',(0.312131472716965,1.21900344770756,0.606078635650713));
#13315=CARTESIAN_POINT('Ctrl Pts',(0.487608314405001,1.28990207050556,-0.000238777108575355));
#13316=CARTESIAN_POINT('Ctrl Pts',(0.497466558273561,1.27931888757273,0.201911276725417));
#13317=CARTESIAN_POINT('Ctrl Pts',(0.507325109482935,1.26873579028159,0.404061320158324));
#13318=CARTESIAN_POINT('Ctrl Pts',(0.517183972542757,1.25815278023897,0.606211353085106));
#13319=CARTESIAN_POINT('Ctrl Pts',(0.693791632045388,1.32642527651154,-0.000115194085079627));
#13320=CARTESIAN_POINT('Ctrl Pts',(0.703280422539661,1.31584113310577,0.202035038813999));
#13321=CARTESIAN_POINT('Ctrl Pts',(0.712769508818955,1.30525706820637,0.404185262036054));
#13322=CARTESIAN_POINT('Ctrl Pts',(0.722258895242942,1.29467308328318,0.606335475483814));
#13323=CARTESIAN_POINT('Ctrl Pts',(0.900000000000002,1.3604297237941,4.33680868994202E-17));
#13324=CARTESIAN_POINT('Ctrl Pts',(0.909119345746935,1.34984469470005,0.202150401646216));
#13325=CARTESIAN_POINT('Ctrl Pts',(0.918238975454289,1.33925973741039,0.40430079432417));
#13326=CARTESIAN_POINT('Ctrl Pts',(0.927358893435711,1.32867485341111,0.606451177918334));
#13327=CARTESIAN_POINT('',(0.313137632044028,1.21919552599286,0.606079286803921));
#13328=CARTESIAN_POINT('Ctrl Pts',(0.900000000000026,1.32415632515176,0.605901073595307));
#13329=CARTESIAN_POINT('Ctrl Pts',(0.703992099548352,1.29143758865737,0.605956720831638));
#13330=CARTESIAN_POINT('Ctrl Pts',(0.508347756773358,1.25646926692181,0.606016122348466));
#13331=CARTESIAN_POINT('Ctrl Pts',(0.313137632044028,1.21919552599286,0.606079286803921));
#13332=CARTESIAN_POINT('Ctrl Pts',(0.313137632044028,1.21919552599286,0.606079286803922));
#13333=CARTESIAN_POINT('Ctrl Pts',(0.302580635585432,1.22970674279184,0.404052833452346));
#13334=CARTESIAN_POINT('Ctrl Pts',(0.29202349034588,1.2402182973453,0.20202640462578));
#13335=CARTESIAN_POINT('Ctrl Pts',(0.28146619846596,1.25073018526678,-6.5594231435373E-18));
#13336=CARTESIAN_POINT('Ctrl Pts',(0.331856371369202,1.12115139781564,0.7));
#13337=CARTESIAN_POINT('Ctrl Pts',(0.526295996270969,1.15827411715321,0.7));
#13338=CARTESIAN_POINT('Ctrl Pts',(0.72117838049967,1.193102781986,0.7));
#13339=CARTESIAN_POINT('Ctrl Pts',(0.916434425702682,1.22569269236154,0.7));
#13340=CARTESIAN_POINT('Ctrl Pts',(0.326462650586141,1.14940237362229,0.699999999999999));
#13341=CARTESIAN_POINT('Ctrl Pts',(0.52112301919326,1.18657973614434,0.700000445015345));
#13342=CARTESIAN_POINT('Ctrl Pts',(0.716221724293519,1.22145811194286,0.699999606692487));
#13343=CARTESIAN_POINT('Ctrl Pts',(0.911693828447618,1.25409504944868,0.700000000000001));
#13344=CARTESIAN_POINT('Ctrl Pts',(0.317109102097967,1.19839394783867,0.676905055067496));
#13345=CARTESIAN_POINT('Ctrl Pts',(0.512149925983836,1.23566412474798,0.676884474751893));
#13346=CARTESIAN_POINT('Ctrl Pts',(0.707628846166824,1.27063023858114,0.676865462359185));
#13347=CARTESIAN_POINT('Ctrl Pts',(0.903473253113193,1.30334701150065,0.676847307332805));
#13348=CARTESIAN_POINT('Ctrl Pts',(0.313383556860882,1.21790743260971,0.627610331402299));
#13349=CARTESIAN_POINT('Ctrl Pts',(0.508581607804839,1.25519230329596,0.627556915196293));
#13350=CARTESIAN_POINT('Ctrl Pts',(0.704212910592822,1.29017057588713,0.627506965865002));
#13351=CARTESIAN_POINT('Ctrl Pts',(0.900209809599685,1.32289929215587,0.627459885485154));
#13352=CARTESIAN_POINT('Ctrl Pts',(0.313137632044028,1.21919552599286,0.606079286803921));
#13353=CARTESIAN_POINT('Ctrl Pts',(0.508347756773358,1.25646926692181,0.606016122348466));
#13354=CARTESIAN_POINT('Ctrl Pts',(0.703992099548352,1.29143758865737,0.605956720831638));
#13355=CARTESIAN_POINT('Ctrl Pts',(0.900000000000026,1.32415632515176,0.605901073595307));
#13356=CARTESIAN_POINT('Origin',(0.3318563713692,1.12115139781563,0.6));
#13357=CARTESIAN_POINT('Origin',(0.3318563713692,1.12115139781563,0.6));
#13358=CARTESIAN_POINT('Origin',(0.3318563713692,1.12115139781563,0.6));
#13359=CARTESIAN_POINT('Origin',(0.331856371369201,1.12115139781563,0.6));
#13360=CARTESIAN_POINT('Origin',(11.6681436286308,1.2964346619681,0.6));
#13361=CARTESIAN_POINT('Origin',(11.6681436286308,1.2964346619681,0.6));
#13362=CARTESIAN_POINT('',(11.7680065821063,1.2964346619681,0.605233595624295));
#13363=CARTESIAN_POINT('Origin',(11.6681436286308,1.2964346619681,0.6));
#13364=CARTESIAN_POINT('Origin',(11.6681436286308,1.2964346619681,0.6));
#13365=CARTESIAN_POINT('Origin',(0.3318563713692,-1.12115139781563,0.6));
#13366=CARTESIAN_POINT('Origin',(0.3318563713692,-1.12115139781563,0.6));
#13367=CARTESIAN_POINT('Origin',(0.3318563713692,-1.12115139781563,0.6));
#13368=CARTESIAN_POINT('Origin',(0.3318563713692,-0.7,0.6));
#13369=CARTESIAN_POINT('Ctrl Pts',(0.281398851089427,-1.25079724300364,
-0.00128877254616805));
#13370=CARTESIAN_POINT('Ctrl Pts',(0.291978592719145,-1.24026300108396,
0.201167222825305));
#13371=CARTESIAN_POINT('Ctrl Pts',(0.302558187088771,-1.2297290939422,0.403623242499903));
#13372=CARTESIAN_POINT('Ctrl Pts',(0.313137632044028,-1.21919552599286,
0.606079286803922));
#13373=CARTESIAN_POINT('Ctrl Pts',(0.258825925396095,-1.24645021448495,
-0.000331836826913007));
#13374=CARTESIAN_POINT('Ctrl Pts',(0.269412087408768,-1.23590982471973,
0.202123507634926));
#13375=CARTESIAN_POINT('Ctrl Pts',(0.279998097240749,-1.22537010804418,
0.404578894752494));
#13376=CARTESIAN_POINT('Ctrl Pts',(0.290584031570127,-1.21483034200885,
0.60703428203898));
#13377=CARTESIAN_POINT('Ctrl Pts',(0.216858515231733,-1.22156435206688,
0.000573427186746937));
#13378=CARTESIAN_POINT('Ctrl Pts',(0.22746089442761,-1.21102065820065,0.20302778119957));
#13379=CARTESIAN_POINT('Ctrl Pts',(0.238063405890532,-1.20047706879609,
0.405482132943502));
#13380=CARTESIAN_POINT('Ctrl Pts',(0.248665715176951,-1.18993398276804,
0.607936521147589));
#13381=CARTESIAN_POINT('Ctrl Pts',(0.20022524016831,-1.1757120364715,-0.000939345874739115));
#13382=CARTESIAN_POINT('Ctrl Pts',(0.210835545796271,-1.16517845930889,
0.201515175954065));
#13383=CARTESIAN_POINT('Ctrl Pts',(0.221445511453644,-1.15464532122135,
0.403969738345816));
#13384=CARTESIAN_POINT('Ctrl Pts',(0.232055819885544,-1.1441124535127,0.606424296559432));
#13385=CARTESIAN_POINT('Ctrl Pts',(0.200162791320387,-1.15273540576203,
-0.00213094087794781));
#13386=CARTESIAN_POINT('Ctrl Pts',(0.210772999146098,-1.14220702337553,
0.200323884929633));
#13387=CARTESIAN_POINT('Ctrl Pts',(0.221383207999129,-1.13167901896849,
0.402778730339676));
#13388=CARTESIAN_POINT('Ctrl Pts',(0.231993417893744,-1.12115139781563,
0.605233595624295));
#13389=CARTESIAN_POINT('Origin',(11.6681436286308,-1.2964346619681,0.6));
#13390=CARTESIAN_POINT('',(11.7680065821063,-1.2964346619681,0.605233595624295));
#13391=CARTESIAN_POINT('Origin',(11.6681436286308,-1.2964346619681,0.6));
#13392=CARTESIAN_POINT('Origin',(11.6681436286308,-1.2964346619681,0.6));
#13393=CARTESIAN_POINT('Origin',(11.6681436286308,0.8,0.6));
#13394=CARTESIAN_POINT('',(11.7680065821063,0.8,0.605233595624295));
#13395=CARTESIAN_POINT('Ctrl Pts',(11.7998406965532,-1.32812796269332,-0.00219749346969486));
#13396=CARTESIAN_POINT('Ctrl Pts',(11.7892293257052,-1.31756329650235,0.200279524124498));
#13397=CARTESIAN_POINT('Ctrl Pts',(11.778617954226,-1.30699886176745,0.402756553762325));
#13398=CARTESIAN_POINT('Ctrl Pts',(11.7680065821063,-1.2964346619681,0.605233595624295));
#13399=CARTESIAN_POINT('Ctrl Pts',(11.7997644051931,-1.35610429277321,-0.000741767599518841));
#13400=CARTESIAN_POINT('Ctrl Pts',(11.7891529352516,-1.34553639595159,0.201735054786578));
#13401=CARTESIAN_POINT('Ctrl Pts',(11.7785417923834,-1.33496887357233,0.404211913913734));
#13402=CARTESIAN_POINT('Ctrl Pts',(11.7679303202531,-1.32440140973518,0.606688758469115));
#13403=CARTESIAN_POINT('Ctrl Pts',(11.777798894316,-1.40464673224301,0.000639873095493681));
#13404=CARTESIAN_POINT('Ctrl Pts',(11.7671928076068,-1.39407357725403,0.203116666245104));
#13405=CARTESIAN_POINT('Ctrl Pts',(11.7565866683578,-1.38350056680667,0.405593463707878));
#13406=CARTESIAN_POINT('Ctrl Pts',(11.7459806329718,-1.37292778989405,0.608070278434593));
#13407=CARTESIAN_POINT('Ctrl Pts',(11.7305637688674,-1.42539741767755,-0.000752904078362463));
#13408=CARTESIAN_POINT('Ctrl Pts',(11.7199663219939,-1.4148278080644,0.201724510929383));
#13409=CARTESIAN_POINT('Ctrl Pts',(11.7093688723049,-1.40425849106451,0.404201940657439));
#13410=CARTESIAN_POINT('Ctrl Pts',(11.6987715660822,-1.39368929079062,0.606679383299034));
#13411=CARTESIAN_POINT('Ctrl Pts',(11.7096810564041,-1.4274931182575,-0.0017379730583696));
#13412=CARTESIAN_POINT('Ctrl Pts',(11.6990862989954,-1.41692678914967,0.200739752511227));
#13413=CARTESIAN_POINT('Ctrl Pts',(11.6884916259906,-1.40636067879325,0.403217493356832));
#13414=CARTESIAN_POINT('Ctrl Pts',(11.6778970386953,-1.39579479040469,0.605695249702977));
#13415=CARTESIAN_POINT('Ctrl Pts',(11.7997255308004,-1.32801330383774,1.58293517182884E-17));
#13416=CARTESIAN_POINT('Ctrl Pts',(11.7891525485321,-1.31748685893698,0.201744519857947));
#13417=CARTESIAN_POINT('Ctrl Pts',(11.7785795656372,-1.30696064383315,0.403489051673192));
#13418=CARTESIAN_POINT('Ctrl Pts',(11.7680065821063,-1.2964346619681,0.605233595624295));
#13419=CARTESIAN_POINT('Ctrl Pts',(11.7096782931395,1.42749036240749,-0.00168516396645821));
#13420=CARTESIAN_POINT('Ctrl Pts',(11.6990844568337,1.41692495195436,0.200774958575157));
#13421=CARTESIAN_POINT('Ctrl Pts',(11.6884907049172,1.40635976021489,0.403235096390144));
#13422=CARTESIAN_POINT('Ctrl Pts',(11.6778970386953,1.39579479040469,0.605695249702978));
#13423=CARTESIAN_POINT('Ctrl Pts',(11.7375219088137,1.42469609383707,-0.000371738767665111));
#13424=CARTESIAN_POINT('Ctrl Pts',(11.7269244310859,1.41412622652679,0.202087962343291));
#13425=CARTESIAN_POINT('Ctrl Pts',(11.7163270893473,1.40355692684423,0.404547700208143));
#13426=CARTESIAN_POINT('Ctrl Pts',(11.7057297418778,1.39298745758592,0.607007427831054));
#13427=CARTESIAN_POINT('Ctrl Pts',(11.7837126264455,1.39812338730171,0.000662527065309348));
#13428=CARTESIAN_POINT('Ctrl Pts',(11.7731059659782,1.38755170250994,0.203121672627585));
#13429=CARTESIAN_POINT('Ctrl Pts',(11.762499302106,1.37698011891703,0.405580822779681));
#13430=CARTESIAN_POINT('Ctrl Pts',(11.7518926781287,1.36640881816393,0.608039989525598));
#13431=CARTESIAN_POINT('Ctrl Pts',(11.7997807104374,1.34910745421534,-0.00105289019631603));
#13432=CARTESIAN_POINT('Ctrl Pts',(11.7891702365097,1.33854134055748,0.201406383632416));
#13433=CARTESIAN_POINT('Ctrl Pts',(11.7785598611315,1.32797539467558,0.403865671186622));
#13434=CARTESIAN_POINT('Ctrl Pts',(11.7679493857164,1.31740972279341,0.60632496775791));
#13435=CARTESIAN_POINT('Ctrl Pts',(11.7998379289556,1.32812520727701,-0.00214468456243374));
#13436=CARTESIAN_POINT('Ctrl Pts',(11.78922748064,1.31756145959839,0.200314730064766));
#13437=CARTESIAN_POINT('Ctrl Pts',(11.7786170316934,1.30699794333589,0.402774156733522));
#13438=CARTESIAN_POINT('Ctrl Pts',(11.7680065821063,1.2964346619681,0.605233595624295));
#13439=CARTESIAN_POINT('Ctrl Pts',(11.7680065821063,1.2964346619681,0.605233595624295));
#13440=CARTESIAN_POINT('Ctrl Pts',(11.7785795656372,1.30696064383315,0.403489051673192));
#13441=CARTESIAN_POINT('Ctrl Pts',(11.7891525485321,1.31748685893698,0.201744519857946));
#13442=CARTESIAN_POINT('Ctrl Pts',(11.7997255308004,1.32801330383774,3.10081821330854E-17));
#13443=CARTESIAN_POINT('Ctrl Pts',(11.3905090053564,1.32332268868375,0.7));
#13444=CARTESIAN_POINT('Ctrl Pts',(11.4830653488871,1.31448403714216,0.7));
#13445=CARTESIAN_POINT('Ctrl Pts',(11.5756099286391,1.3055179747114,0.7));
#13446=CARTESIAN_POINT('Ctrl Pts',(11.6681436286308,1.2964346619681,0.7));
#13447=CARTESIAN_POINT('Ctrl Pts',(11.3932507170007,1.35203326785047,0.7));
#13448=CARTESIAN_POINT('Ctrl Pts',(11.4858332859074,1.34318985044544,0.699999917777441));
#13449=CARTESIAN_POINT('Ctrl Pts',(11.5784027531871,1.33421922733773,0.700000082825348));
#13450=CARTESIAN_POINT('Ctrl Pts',(11.6709605510772,1.32513126902304,0.7));
#13451=CARTESIAN_POINT('Ctrl Pts',(11.3980029235658,1.40179729139028,0.67675176769038));
#13452=CARTESIAN_POINT('Ctrl Pts',(11.4906306781252,1.39294591144353,0.676755553516685));
#13453=CARTESIAN_POINT('Ctrl Pts',(11.583243842395,1.38396722707511,0.676759299309383));
#13454=CARTESIAN_POINT('Ctrl Pts',(11.6758431636759,1.37487151491717,0.676763114282959));
#13455=CARTESIAN_POINT('Ctrl Pts',(11.3998836071583,1.4214913811319,0.627256563056779));
#13456=CARTESIAN_POINT('Ctrl Pts',(11.4925297866457,1.41264104586547,0.627266369072496));
#13457=CARTESIAN_POINT('Ctrl Pts',(11.5851604051362,1.40366358810601,0.627276165220861));
#13458=CARTESIAN_POINT('Ctrl Pts',(11.6777767156198,1.39456903283364,0.627286048421068));
#13459=CARTESIAN_POINT('Ctrl Pts',(11.4,1.4227102204299,0.605660349289938));
#13460=CARTESIAN_POINT('Ctrl Pts',(11.4926474653491,1.41386220753305,0.605671932550561));
#13461=CARTESIAN_POINT('Ctrl Pts',(11.585279512325,1.40488700096013,0.605683574233495));
#13462=CARTESIAN_POINT('Ctrl Pts',(11.6778970386953,1.39579479040469,0.605695249702977));
#13463=CARTESIAN_POINT('Ctrl Pts',(0.200160078391861,1.15273809776858,-0.00218270663797729));
#13464=CARTESIAN_POINT('Ctrl Pts',(0.210771190526905,1.14220881798213,0.200289374419605));
#13465=CARTESIAN_POINT('Ctrl Pts',(0.221382303689445,1.13167991623912,0.402761475082968));
#13466=CARTESIAN_POINT('Ctrl Pts',(0.231993417893744,1.12115139781563,0.605233595624295));
#13467=CARTESIAN_POINT('Ctrl Pts',(0.200222527243758,1.17571472979894,-0.000991111558954063));
#13468=CARTESIAN_POINT('Ctrl Pts',(0.210833737189325,1.165180254798,0.201480665494204));
#13469=CARTESIAN_POINT('Ctrl Pts',(0.22144460713556,1.15464621893915,0.403952483115279));
#13470=CARTESIAN_POINT('Ctrl Pts',(0.232055819885544,1.1441124535127,0.606424296559433));
#13471=CARTESIAN_POINT('Ctrl Pts',(0.216855804290742,1.22156704800519,0.000521661548984882));
#13472=CARTESIAN_POINT('Ctrl Pts',(0.22745908713481,1.21102245544698,0.202993270772045));
#13473=CARTESIAN_POINT('Ctrl Pts',(0.238062502254218,1.2004779673848,0.405464877727456));
#13474=CARTESIAN_POINT('Ctrl Pts',(0.248665715176951,1.18993398276804,0.607936521147589));
#13475=CARTESIAN_POINT('Ctrl Pts',(0.258823218619159,1.24645290953083,-0.000383602721372307));
#13476=CARTESIAN_POINT('Ctrl Pts',(0.269410282911183,1.23591162135389,0.202088997034388));
#13477=CARTESIAN_POINT('Ctrl Pts',(0.279997195000074,1.22537100634993,0.404561639451295));
#13478=CARTESIAN_POINT('Ctrl Pts',(0.290584031570127,1.21483034200885,0.60703428203898));
#13479=CARTESIAN_POINT('Ctrl Pts',(0.281396145950812,1.25079993650842,-0.00134053860524368));
#13480=CARTESIAN_POINT('Ctrl Pts',(0.291976789318506,1.24026479669674,0.201132712115111));
#13481=CARTESIAN_POINT('Ctrl Pts',(0.302557285401186,1.22972999171968,0.403605987142707));
#13482=CARTESIAN_POINT('Ctrl Pts',(0.313137632044028,1.21919552599286,0.606079286803922));
#13483=CARTESIAN_POINT('Origin',(11.8002740930491,1.6,-0.0104671912485888));
#13484=CARTESIAN_POINT('Origin',(0.3318563713692,1.12115139781563,0.6));
#13485=CARTESIAN_POINT('',(0.331856371369203,1.12115139781563,0.9));
#13486=CARTESIAN_POINT('',(0.0322675109428288,1.12115139781563,0.615700786872883));
#13487=CARTESIAN_POINT('Origin',(0.3318563713692,1.12115139781563,0.6));
#13488=CARTESIAN_POINT('',(0.275700153393682,1.4152837823473,0.618237860411764));
#13489=CARTESIAN_POINT('Origin',(0.3318563713692,1.12115139781563,0.6));
#13490=CARTESIAN_POINT('Origin',(0.331856371369201,1.12115139781563,0.600000000000001));
#13491=CARTESIAN_POINT('Origin',(11.6681436286308,1.2964346619681,0.6));
#13492=CARTESIAN_POINT('',(11.6681436286308,1.2964346619681,0.9));
#13493=CARTESIAN_POINT('',(11.6974038588243,1.59451504727786,0.617085749108931));
#13494=CARTESIAN_POINT('Origin',(11.6681436286308,1.2964346619681,0.6));
#13495=CARTESIAN_POINT('',(11.9677324890572,1.2964346619681,0.615700786872884));
#13496=CARTESIAN_POINT('Origin',(11.6681436286308,1.2964346619681,0.6));
#13497=CARTESIAN_POINT('Origin',(11.6681436286308,1.2964346619681,0.6));
#13498=CARTESIAN_POINT('Origin',(0.3318563713692,-1.12115139781563,0.6));
#13499=CARTESIAN_POINT('',(0.3318563713692,-1.12115139781563,0.9));
#13500=CARTESIAN_POINT('',(0.27570015339368,-1.4152837823473,0.618237860411764));
#13501=CARTESIAN_POINT('Origin',(0.331856371369206,-1.12115139781563,0.6));
#13502=CARTESIAN_POINT('',(0.0322675109428289,-1.12115139781563,0.615700786872884));
#13503=CARTESIAN_POINT('Origin',(0.3318563713692,-1.12115139781563,0.6));
#13504=CARTESIAN_POINT('Origin',(0.331856371369201,-1.12115139781563,0.6));
#13505=CARTESIAN_POINT('Origin',(0.3318563713692,-0.7,0.6));
#13506=CARTESIAN_POINT('',(0.0322675109428288,-0.7,0.615700786872883));
#13507=CARTESIAN_POINT('',(0.3318563713692,-0.7,0.9));
#13508=CARTESIAN_POINT('Ctrl Pts',(0.243379792658812,-1.44768816351885,
-0.00386660544379547));
#13509=CARTESIAN_POINT('Ctrl Pts',(0.254153714020244,-1.43688644166428,
0.203501514337738));
#13510=CARTESIAN_POINT('Ctrl Pts',(0.264927169923045,-1.42608498030896,
0.410869669467268));
#13511=CARTESIAN_POINT('Ctrl Pts',(0.275700153393682,-1.4152837823473,0.618237860411764));
#13512=CARTESIAN_POINT('Ctrl Pts',(0.165985306518657,-1.43278556900406,
-0.000585522405354874));
#13513=CARTESIAN_POINT('Ctrl Pts',(0.176781886982148,-1.42196211044871,
0.206780297826791));
#13514=CARTESIAN_POINT('Ctrl Pts',(0.187577631459021,-1.41114055376332,
0.414146260476818));
#13515=CARTESIAN_POINT('Ctrl Pts',(0.198373523197449,-1.40031743725927,
0.621512129789107));
#13516=CARTESIAN_POINT('Ctrl Pts',(0.0420337764471552,-1.35067831466576,
0.00164062070145552));
#13517=CARTESIAN_POINT('Ctrl Pts',(0.0528811856485653,-1.33984924001505,
0.209003590924217));
#13518=CARTESIAN_POINT('Ctrl Pts',(0.0637288270387668,-1.3290196870647,
0.416366521726085));
#13519=CARTESIAN_POINT('Ctrl Pts',(0.0745760486629849,-1.31819094697801,
0.623729515932473));
#13520=CARTESIAN_POINT('Ctrl Pts',(-0.000174449685670057,-1.21258510413485,
-0.00332869829739982));
#13521=CARTESIAN_POINT('Ctrl Pts',(0.0106931634330696,-1.20178787588112,
0.204035045544629));
#13522=CARTESIAN_POINT('Ctrl Pts',(0.0215603573327632,-1.19099068058357,
0.411398812224037));
#13523=CARTESIAN_POINT('Ctrl Pts',(0.0324279732074593,-1.18019411246525,
0.618762589277523));
#13524=CARTESIAN_POINT('Ctrl Pts',(-0.000335035344191381,-1.15350137313465,
-0.00639285519773308));
#13525=CARTESIAN_POINT('Ctrl Pts',(0.0105324790023165,-1.1427176497384,
0.200971671503832));
#13526=CARTESIAN_POINT('Ctrl Pts',(0.0213999944262164,-1.13193432274319,
0.408336218763261));
#13527=CARTESIAN_POINT('Ctrl Pts',(0.0322675109428286,-1.12115139781563,
0.615700786872884));
#13528=CARTESIAN_POINT('Ctrl Pts',(0.243580684154575,-1.44748675362873,
-2.16840434497101E-17));
#13529=CARTESIAN_POINT('Ctrl Pts',(0.254287635915809,-1.43675217163244,
0.206079251738322));
#13530=CARTESIAN_POINT('Ctrl Pts',(0.264994127943615,-1.42601784692504,
0.412158538389471));
#13531=CARTESIAN_POINT('Ctrl Pts',(0.275700153393682,-1.4152837823473,0.618237860411764));
#13532=CARTESIAN_POINT('Ctrl Pts',(0.0322675109428286,-1.12115139781563,
0.615700786872884));
#13533=CARTESIAN_POINT('Ctrl Pts',(0.0215116728964671,-1.13182351356624,
0.410467170919192));
#13534=CARTESIAN_POINT('Ctrl Pts',(0.0107558359204751,-1.14249602316337,
0.205233575389367));
#13535=CARTESIAN_POINT('Ctrl Pts',(-1.41190227911925E-16,-1.15316892111333,
8.06646416329215E-17));
#13536=CARTESIAN_POINT('Origin',(11.6681436286308,-1.2964346619681,0.6));
#13537=CARTESIAN_POINT('',(11.9677324890572,-1.2964346619681,0.615700786872884));
#13538=CARTESIAN_POINT('',(11.6974038588243,-1.59451504727786,0.617085749108931));
#13539=CARTESIAN_POINT('Origin',(11.6681436286308,-1.2964346619681,0.600000000000001));
#13540=CARTESIAN_POINT('',(11.6681436286308,-1.2964346619681,0.9));
#13541=CARTESIAN_POINT('Origin',(11.6681436286308,-1.2964346619681,0.6));
#13542=CARTESIAN_POINT('Origin',(11.6681436286308,-1.2964346619681,0.6));
#13543=CARTESIAN_POINT('Origin',(11.6681436286308,0.8,0.6));
#13544=CARTESIAN_POINT('',(11.9677324890572,0.8,0.615700786872884));
#13545=CARTESIAN_POINT('',(11.6681436286308,0.8,0.9));
#13546=CARTESIAN_POINT('Ctrl Pts',(11.6681436286308,-1.2964346619681,0.9));
#13547=CARTESIAN_POINT('Ctrl Pts',(10.0505146497799,-1.45522470190849,0.9));
#13548=CARTESIAN_POINT('Ctrl Pts',(7.34698379851713,-1.66064017564263,0.9));
#13549=CARTESIAN_POINT('Ctrl Pts',(3.5507249968367,-1.5921338472202,0.9));
#13550=CARTESIAN_POINT('Ctrl Pts',(1.39628032950236,-1.32437289587156,0.9));
#13551=CARTESIAN_POINT('Ctrl Pts',(0.331856371369199,-1.12115139781563,
0.9));
#13552=CARTESIAN_POINT('Ctrl Pts',(11.6765943959699,-1.38252448313292,0.9));
#13553=CARTESIAN_POINT('Ctrl Pts',(10.0577014803155,-1.54155822929668,0.900004386952174));
#13554=CARTESIAN_POINT('Ctrl Pts',(7.35045927226653,-1.74750661992774,0.90000020513805));
#13555=CARTESIAN_POINT('Ctrl Pts',(3.54497585078588,-1.67885197560093,0.899998846478116));
#13556=CARTESIAN_POINT('Ctrl Pts',(1.38372480803625,-1.41002339692611,0.900007381454799));
#13557=CARTESIAN_POINT('Ctrl Pts',(0.315675209020016,-1.2059043252356,0.9));
#13558=CARTESIAN_POINT('Ctrl Pts',(11.6912432102654,-1.53175516862908,0.830242007927396));
#13559=CARTESIAN_POINT('Ctrl Pts',(10.070172518288,-1.69119563674726,0.830042231904815));
#13560=CARTESIAN_POINT('Ctrl Pts',(7.35645297288469,-1.89806162871739,0.829725685238203));
#13561=CARTESIAN_POINT('Ctrl Pts',(3.53503777381493,-1.8291593714544,0.829829026055289));
#13562=CARTESIAN_POINT('Ctrl Pts',(1.36192166831068,-1.55847530615989,0.830279056498203));
#13563=CARTESIAN_POINT('Ctrl Pts',(0.28762358730286,-1.35283178372728,0.830616544072481));
#13564=CARTESIAN_POINT('Ctrl Pts',(11.6970428895979,-1.59083777456472,0.681858145263203));
#13565=CARTESIAN_POINT('Ctrl Pts',(10.0750816081461,-1.75021732245097,0.681339641080976));
#13566=CARTESIAN_POINT('Ctrl Pts',(7.3588078744758,-1.95708146899443,0.680519979048775));
#13567=CARTESIAN_POINT('Ctrl Pts',(3.53113644431293,-1.88819699008302,0.68078748362792));
#13568=CARTESIAN_POINT('Ctrl Pts',(1.35331700817769,-1.61730376958615,0.681953432622034));
#13569=CARTESIAN_POINT('Ctrl Pts',(0.276437927844241,-1.41141950219787,
0.682830994206899));
#13570=CARTESIAN_POINT('Ctrl Pts',(11.6974038588243,-1.59451504727786,0.617085749108931));
#13571=CARTESIAN_POINT('Ctrl Pts',(10.0753786444688,-1.75377172884558,0.616473434532366));
#13572=CARTESIAN_POINT('Ctrl Pts',(7.35893161235257,-1.96044797105896,0.61550283428964));
#13573=CARTESIAN_POINT('Ctrl Pts',(3.53092277948893,-1.89162724517065,0.615818637525046));
#13574=CARTESIAN_POINT('Ctrl Pts',(1.35277799022997,-1.62098550016515,0.617200513836093));
#13575=CARTESIAN_POINT('Ctrl Pts',(0.27570015339368,-1.4152837823473,0.618237860411764));
#13576=CARTESIAN_POINT('Ctrl Pts',(0.27570015339368,-1.4152837823473,0.618237860411764));
#13577=CARTESIAN_POINT('Ctrl Pts',(1.35277799022997,-1.62098550016515,0.617200513836093));
#13578=CARTESIAN_POINT('Ctrl Pts',(3.53092277948893,-1.89162724517065,0.615818637525046));
#13579=CARTESIAN_POINT('Ctrl Pts',(7.35893161235257,-1.96044797105896,0.61550283428964));
#13580=CARTESIAN_POINT('Ctrl Pts',(10.0753786444688,-1.75377172884558,0.616473434532366));
#13581=CARTESIAN_POINT('Ctrl Pts',(11.6974038588243,-1.59451504727786,0.617085749108931));
#13582=CARTESIAN_POINT('Ctrl Pts',(11.6681436286308,-1.2964346619681,0.9));
#13583=CARTESIAN_POINT('Ctrl Pts',(10.0505146497799,-1.45522470190849,0.9));
#13584=CARTESIAN_POINT('Ctrl Pts',(7.34698379851713,-1.66064017564263,0.9));
#13585=CARTESIAN_POINT('Ctrl Pts',(3.5507249968367,-1.5921338472202,0.9));
#13586=CARTESIAN_POINT('Ctrl Pts',(1.39628032950236,-1.32437289587156,0.9));
#13587=CARTESIAN_POINT('Ctrl Pts',(0.331856371369199,-1.12115139781563,
0.9));
#13588=CARTESIAN_POINT('Ctrl Pts',(12.0003454972153,-1.32890342861544,-0.00659247958978532));
#13589=CARTESIAN_POINT('Ctrl Pts',(11.9894744951615,-1.31808026232082,0.200838596530835));
#13590=CARTESIAN_POINT('Ctrl Pts',(11.9786034924455,-1.30725733885828,0.408269685287046));
#13591=CARTESIAN_POINT('Ctrl Pts',(11.9677324890572,-1.2964346619681,0.615700786872884));
#13592=CARTESIAN_POINT('Ctrl Pts',(12.000116620981,-1.41283311850955,-0.00222526087931226));
#13593=CARTESIAN_POINT('Ctrl Pts',(11.9892453109784,-1.40200002127642,0.205205215027088));
#13594=CARTESIAN_POINT('Ctrl Pts',(11.9783750177566,-1.39116761830557,0.412635780645844));
#13595=CARTESIAN_POINT('Ctrl Pts',(11.9675037034976,-1.38033490526933,0.620066275407343));
#13596=CARTESIAN_POINT('Ctrl Pts',(11.9341774721098,-1.5584705948029,0.00191796595980313));
#13597=CARTESIAN_POINT('Ctrl Pts',(11.9233226835938,-1.54762133657986,0.209348350794306));
#13598=CARTESIAN_POINT('Ctrl Pts',(11.9124678718222,-1.53677206634062,0.416778732304926));
#13599=CARTESIAN_POINT('Ctrl Pts',(11.9016132473252,-1.52592301942363,0.624209134118803));
#13600=CARTESIAN_POINT('Ctrl Pts',(11.7925116537096,-1.62071287545028,-0.0022587989925734));
#13601=CARTESIAN_POINT('Ctrl Pts',(11.7816834491585,-1.6098745265243,0.205173499361722));
#13602=CARTESIAN_POINT('Ctrl Pts',(11.7708551999607,-1.59903658749835,0.41260581547062));
#13603=CARTESIAN_POINT('Ctrl Pts',(11.760027440985,-1.58819854843564,0.620038149897102));
#13604=CARTESIAN_POINT('Ctrl Pts',(11.7298629188572,-1.62699926142283,-0.0052140742384003));
#13605=CARTESIAN_POINT('Ctrl Pts',(11.7190429637906,-1.61617098622686,0.202219177289036));
#13606=CARTESIAN_POINT('Ctrl Pts',(11.708223275703,-1.60534291388117,0.409652451626141));
#13607=CARTESIAN_POINT('Ctrl Pts',(11.6974038588243,-1.59451504727786,0.617085749108931));
#13608=CARTESIAN_POINT('Ctrl Pts',(12.,-1.32855945177638,-1.94722710178397E-16));
#13609=CARTESIAN_POINT('Ctrl Pts',(11.9892441636707,-1.31785094954632,0.205233583190348));
#13610=CARTESIAN_POINT('Ctrl Pts',(11.978488326693,-1.30714268506935,0.410467178751997));
#13611=CARTESIAN_POINT('Ctrl Pts',(11.9677324890572,-1.2964346619681,0.615700786872884));
#13612=CARTESIAN_POINT('Ctrl Pts',(11.6974038588243,-1.59451504727786,0.617085749108931));
#13613=CARTESIAN_POINT('Ctrl Pts',(11.7081326228587,-1.605252190239,0.41139047675572));
#13614=CARTESIAN_POINT('Ctrl Pts',(11.7188616535763,-1.61598953550924,0.205695227161956));
#13615=CARTESIAN_POINT('Ctrl Pts',(11.7295909468525,-1.62672708026858,8.73866951023317E-17));
#13616=CARTESIAN_POINT('Ctrl Pts',(11.7298546566854,1.62699099289774,-0.00505567716946009));
#13617=CARTESIAN_POINT('Ctrl Pts',(11.719037455812,1.61616547398006,0.202324775346606));
#13618=CARTESIAN_POINT('Ctrl Pts',(11.7082205217827,1.60534015781013,0.409705250660816));
#13619=CARTESIAN_POINT('Ctrl Pts',(11.6974038588243,1.59451504727786,0.617085749108931));
#13620=CARTESIAN_POINT('Ctrl Pts',(11.8133862946664,1.61860913476435,-0.00111531114554236));
#13621=CARTESIAN_POINT('Ctrl Pts',(11.8025579038448,1.6077699189899,0.206263846261978));
#13622=CARTESIAN_POINT('Ctrl Pts',(11.7917299466398,1.59693199028804,0.41364309356145));
#13623=CARTESIAN_POINT('Ctrl Pts',(11.7809019683719,1.58609304882157,0.621022283493159));
#13624=CARTESIAN_POINT('Ctrl Pts',(11.9519653779615,1.53884931758497,0.00198566945999789));
#13625=CARTESIAN_POINT('Ctrl Pts',(11.9411087765487,1.52800449744246,0.209363119024413));
#13626=CARTESIAN_POINT('Ctrl Pts',(11.9302521502216,1.51715965702667,0.416740564833343));
#13627=CARTESIAN_POINT('Ctrl Pts',(11.9193956662674,1.50631506689811,0.624118030142866));
#13628=CARTESIAN_POINT('Ctrl Pts',(12.0001655389052,1.39184242582033,-0.00315867047762133));
#13629=CARTESIAN_POINT('Ctrl Pts',(11.9892972278067,1.38101476165208,0.204219175612729));
#13630=CARTESIAN_POINT('Ctrl Pts',(11.9784292129672,1.37018709651964,0.41159703650799));
#13631=CARTESIAN_POINT('Ctrl Pts',(11.9675608998875,1.35935984444403,0.618974903273729));
#13632=CARTESIAN_POINT('Ctrl Pts',(12.0003371960637,1.32889516399154,-0.00643408418199817));
#13633=CARTESIAN_POINT('Ctrl Pts',(11.9894689610601,1.31807475269516,0.200944193475792));
#13634=CARTESIAN_POINT('Ctrl Pts',(11.9786007253947,1.3072545841082,0.408322483762789));
#13635=CARTESIAN_POINT('Ctrl Pts',(11.9677324890572,1.2964346619681,0.615700786872884));
#13636=CARTESIAN_POINT('Ctrl Pts',(11.7295909468525,1.62672708026857,-8.50014503228635E-17));
#13637=CARTESIAN_POINT('Ctrl Pts',(11.7188616535763,1.61598953550924,0.205695227161956));
#13638=CARTESIAN_POINT('Ctrl Pts',(11.7081326228587,1.605252190239,0.411390476755719));
#13639=CARTESIAN_POINT('Ctrl Pts',(11.6974038588243,1.59451504727786,0.617085749108931));
#13640=CARTESIAN_POINT('Ctrl Pts',(11.9677324890572,1.2964346619681,0.615700786872884));
#13641=CARTESIAN_POINT('Ctrl Pts',(11.978488326693,1.30714268506935,0.410467178751997));
#13642=CARTESIAN_POINT('Ctrl Pts',(11.9892441636707,1.31785094954633,0.205233583190349));
#13643=CARTESIAN_POINT('Ctrl Pts',(12.,1.32855945177638,-2.38524477946811E-17));
#13644=CARTESIAN_POINT('Ctrl Pts',(0.3318563713692,1.12115139781563,0.9));
#13645=CARTESIAN_POINT('Ctrl Pts',(1.92849230856897,1.42598364489954,0.9));
#13646=CARTESIAN_POINT('Ctrl Pts',(5.71993880054687,1.76935652211139,0.9));
#13647=CARTESIAN_POINT('Ctrl Pts',(9.51130499016288,1.50815471522196,0.9));
#13648=CARTESIAN_POINT('Ctrl Pts',(11.6681436286308,1.2964346619681,0.9));
#13649=CARTESIAN_POINT('Ctrl Pts',(0.315675209020018,1.2059043252356,0.9));
#13650=CARTESIAN_POINT('Ctrl Pts',(1.91774960754439,1.51208293277137,0.900011072182198));
#13651=CARTESIAN_POINT('Ctrl Pts',(5.72069615836457,1.85663493780214,0.899990666655967));
#13652=CARTESIAN_POINT('Ctrl Pts',(9.5180705084307,1.59456947801794,0.900005849269565));
#13653=CARTESIAN_POINT('Ctrl Pts',(11.6765943959699,1.38252448313292,0.9));
#13654=CARTESIAN_POINT('Ctrl Pts',(0.287623587302861,1.35283178372728,0.83061654407248));
#13655=CARTESIAN_POINT('Ctrl Pts',(1.89907070881462,1.6612970673762,0.830110312711064));
#13656=CARTESIAN_POINT('Ctrl Pts',(5.72203120258494,2.00791989451774,0.829536565111056));
#13657=CARTESIAN_POINT('Ctrl Pts',(9.52981562096212,1.74434245945332,0.829975639897288));
#13658=CARTESIAN_POINT('Ctrl Pts',(11.6912432102654,1.53175516862908,0.830242007927395));
#13659=CARTESIAN_POINT('Ctrl Pts',(0.276437927844243,1.41141950219787,0.682830994206899));
#13660=CARTESIAN_POINT('Ctrl Pts',(1.89175654834445,1.7202459032803,0.681514651829601));
#13661=CARTESIAN_POINT('Ctrl Pts',(5.72254254462207,2.06699613896002,0.680031275065471));
#13662=CARTESIAN_POINT('Ctrl Pts',(9.53442784766217,1.80334383841306,0.681166806353567));
#13663=CARTESIAN_POINT('Ctrl Pts',(11.6970428895979,1.59083777456472,0.681858145263204));
#13664=CARTESIAN_POINT('Ctrl Pts',(0.275700153393682,1.4152837823473,0.618237860411764));
#13665=CARTESIAN_POINT('Ctrl Pts',(1.89131690864814,1.72383635907408,0.616681840548257));
#13666=CARTESIAN_POINT('Ctrl Pts',(5.72257555688819,2.07025489722917,0.614922376024419));
#13667=CARTESIAN_POINT('Ctrl Pts',(9.53470357301702,1.80685728936816,0.616269329673511));
#13668=CARTESIAN_POINT('Ctrl Pts',(11.6974038588243,1.59451504727786,0.617085749108931));
#13669=CARTESIAN_POINT('Ctrl Pts',(11.6974038588243,1.59451504727786,0.617085749108931));
#13670=CARTESIAN_POINT('Ctrl Pts',(9.53470357301702,1.80685728936816,0.616269329673511));
#13671=CARTESIAN_POINT('Ctrl Pts',(5.72257555688819,2.07025489722917,0.614922376024419));
#13672=CARTESIAN_POINT('Ctrl Pts',(1.89131690864814,1.72383635907408,0.616681840548257));
#13673=CARTESIAN_POINT('Ctrl Pts',(0.275700153393682,1.4152837823473,0.618237860411764));
#13674=CARTESIAN_POINT('Ctrl Pts',(0.3318563713692,1.12115139781563,0.9));
#13675=CARTESIAN_POINT('Ctrl Pts',(1.92849230856897,1.42598364489954,0.9));
#13676=CARTESIAN_POINT('Ctrl Pts',(5.71993880054687,1.76935652211139,0.9));
#13677=CARTESIAN_POINT('Ctrl Pts',(9.51130499016288,1.50815471522196,0.9));
#13678=CARTESIAN_POINT('Ctrl Pts',(11.6681436286308,1.2964346619681,0.9));
#13679=CARTESIAN_POINT('Ctrl Pts',(-0.000343174493958709,1.15350944952984,
-0.00654815942696785));
#13680=CARTESIAN_POINT('Ctrl Pts',(0.0105270529019337,1.14272303380391,
0.200868135340743));
#13681=CARTESIAN_POINT('Ctrl Pts',(0.0213972813757523,1.13193701467556,
0.408284450676511));
#13682=CARTESIAN_POINT('Ctrl Pts',(0.0322675109428289,1.12115139781563,
0.615700786872884));
#13683=CARTESIAN_POINT('Ctrl Pts',(-0.000129060241737355,1.23228777111366,
-0.0024626161135415));
#13684=CARTESIAN_POINT('Ctrl Pts',(0.0107416412387167,1.22148297235423,
0.204952596860618));
#13685=CARTESIAN_POINT('Ctrl Pts',(0.0216107531875107,1.21067920461451,
0.412367946918899));
#13686=CARTESIAN_POINT('Ctrl Pts',(0.0324814606290031,1.19987501734845,
0.61978319007907));
#13687=CARTESIAN_POINT('Ctrl Pts',(0.0574602827844584,1.36931747586956,
0.00164530659801973));
#13688=CARTESIAN_POINT('Ctrl Pts',(0.0683025556324749,1.35848226928888,
0.209060253413207));
#13689=CARTESIAN_POINT('Ctrl Pts',(0.079145272670006,1.34764679267913,0.416475160658282));
#13690=CARTESIAN_POINT('Ctrl Pts',(0.0899872847341513,1.33681188280878,
0.62389013300849));
#13691=CARTESIAN_POINT('Ctrl Pts',(0.185325846363896,1.43651931939441,-0.00156109881554352));
#13692=CARTESIAN_POINT('Ctrl Pts',(0.196119220517603,1.4256988926218,0.205857093047737));
#13693=CARTESIAN_POINT('Ctrl Pts',(0.20691256009293,1.41487906031557,0.413275315721495));
#13694=CARTESIAN_POINT('Ctrl Pts',(0.217705180746507,1.40405902353128,0.620693562444772));
#13695=CARTESIAN_POINT('Ctrl Pts',(0.243371723604776,1.44769625339383,-0.00402191236404));
#13696=CARTESIAN_POINT('Ctrl Pts',(0.254148334883323,1.43689183478419,0.203397976373256));
#13697=CARTESIAN_POINT('Ctrl Pts',(0.264924480472538,1.42608767680315,0.410817900476086));
#13698=CARTESIAN_POINT('Ctrl Pts',(0.275700153393682,1.4152837823473,0.618237860411764));
#13699=CARTESIAN_POINT('Ctrl Pts',(-1.23734572934908E-17,1.15316892111333,
-8.67361737988404E-19));
#13700=CARTESIAN_POINT('Ctrl Pts',(0.0107558359204753,1.14249602316336,
0.205233575389367));
#13701=CARTESIAN_POINT('Ctrl Pts',(0.0215116728964674,1.13182351356624,
0.410467170919192));
#13702=CARTESIAN_POINT('Ctrl Pts',(0.0322675109428289,1.12115139781563,
0.615700786872884));
#13703=CARTESIAN_POINT('Ctrl Pts',(0.275700153393682,1.4152837823473,0.618237860411764));
#13704=CARTESIAN_POINT('Ctrl Pts',(0.264994127943615,1.42601784692504,0.412158538389472));
#13705=CARTESIAN_POINT('Ctrl Pts',(0.254287635915814,1.43675217163244,0.206079251738322));
#13706=CARTESIAN_POINT('Ctrl Pts',(0.243580684154575,1.44748675362873,-1.9298798670242E-17));
#13707=CARTESIAN_POINT('Ctrl Pts',(11.7295909468525,-1.62672708026858,0.));
#13708=CARTESIAN_POINT('Ctrl Pts',(11.7192775324813,-1.61592692249094,0.206079286804135));
#13709=CARTESIAN_POINT('Ctrl Pts',(11.70896411811,-1.6051267647133,0.41215857360827));
#13710=CARTESIAN_POINT('Ctrl Pts',(11.6986507037388,-1.59432660693566,0.618237860412405));
#13711=CARTESIAN_POINT('Ctrl Pts',(7.90092085928651,-2.00057770191527,0.));
#13712=CARTESIAN_POINT('Ctrl Pts',(7.89749915175266,-1.98977754413763,0.206079286804135));
#13713=CARTESIAN_POINT('Ctrl Pts',(7.89407744421881,-1.97897738636,0.41215857360827));
#13714=CARTESIAN_POINT('Ctrl Pts',(7.89065573668496,-1.96817722858236,0.618237860412405));
#13715=CARTESIAN_POINT('Ctrl Pts',(4.07225077172054,-2.17467835246083,0.));
#13716=CARTESIAN_POINT('Ctrl Pts',(4.07572077102407,-2.16387819468319,0.206079286804135));
#13717=CARTESIAN_POINT('Ctrl Pts',(4.07919077032759,-2.15307803690555,0.41215857360827));
#13718=CARTESIAN_POINT('Ctrl Pts',(4.08266076963111,-2.14227787912792,0.618237860412405));
#13719=CARTESIAN_POINT('Ctrl Pts',(0.243580684154574,-1.44748675362873,
0.));
#13720=CARTESIAN_POINT('Ctrl Pts',(0.253942390295469,-1.43668659585109,
0.206079286804135));
#13721=CARTESIAN_POINT('Ctrl Pts',(0.264304096436365,-1.42588643807345,
0.41215857360827));
#13722=CARTESIAN_POINT('Ctrl Pts',(0.27466580257726,-1.41508628029581,0.618237860412405));
#13723=CARTESIAN_POINT('Origin',(0.,-1.4,0.));
#13724=CARTESIAN_POINT('Origin',(6.08012166120517,1.06803409199199E-16,
0.9));
#13725=CARTESIAN_POINT('Ctrl Pts',(0.243580684154574,1.44748675362873,0.));
#13726=CARTESIAN_POINT('Ctrl Pts',(0.253942390295469,1.43668659585109,0.206079286804135));
#13727=CARTESIAN_POINT('Ctrl Pts',(0.264304096436365,1.42588643807345,0.41215857360827));
#13728=CARTESIAN_POINT('Ctrl Pts',(0.27466580257726,1.41508628029581,0.618237860412405));
#13729=CARTESIAN_POINT('Ctrl Pts',(4.07225077172054,2.17467835246083,0.));
#13730=CARTESIAN_POINT('Ctrl Pts',(4.07572077102407,2.16387819468319,0.206079286804135));
#13731=CARTESIAN_POINT('Ctrl Pts',(4.07919077032759,2.15307803690555,0.41215857360827));
#13732=CARTESIAN_POINT('Ctrl Pts',(4.08266076963111,2.14227787912792,0.618237860412405));
#13733=CARTESIAN_POINT('Ctrl Pts',(7.90092085928651,2.00057770191527,0.));
#13734=CARTESIAN_POINT('Ctrl Pts',(7.89749915175266,1.98977754413763,0.206079286804135));
#13735=CARTESIAN_POINT('Ctrl Pts',(7.89407744421881,1.97897738636,0.41215857360827));
#13736=CARTESIAN_POINT('Ctrl Pts',(7.89065573668496,1.96817722858236,0.618237860412405));
#13737=CARTESIAN_POINT('Ctrl Pts',(11.7295909468525,1.62672708026858,0.));
#13738=CARTESIAN_POINT('Ctrl Pts',(11.7192775324813,1.61592692249094,0.206079286804135));
#13739=CARTESIAN_POINT('Ctrl Pts',(11.70896411811,1.6051267647133,0.41215857360827));
#13740=CARTESIAN_POINT('Ctrl Pts',(11.6986507037388,1.59432660693566,0.618237860412405));
#13741=CARTESIAN_POINT('Origin',(12.,1.6,0.));
#19453=UNCERTAINTY_MEASURE_WITH_UNIT(LENGTH_MEASURE(0.001),#19472,
'DISTANCE_ACCURACY_VALUE',
'Maximum model space distance between geometric entities at asserted c
onnectivities');
#19458=UNCERTAINTY_MEASURE_WITH_UNIT(LENGTH_MEASURE(0.001),#19472,
'DISTANCE_ACCURACY_VALUE',
'Maximum model space distance between geometric entities at asserted c
onnectivities');
#19466=(
GEOMETRIC_REPRESENTATION_CONTEXT(3)
GLOBAL_UNCERTAINTY_ASSIGNED_CONTEXT((#19453))
GLOBAL_UNIT_ASSIGNED_CONTEXT((#19472,#19474,#19475))
REPRESENTATION_CONTEXT('','3D')
);
#19471=(
GEOMETRIC_REPRESENTATION_CONTEXT(3)
GLOBAL_UNCERTAINTY_ASSIGNED_CONTEXT((#19458))
GLOBAL_UNIT_ASSIGNED_CONTEXT((#19472,#19474,#19475))
REPRESENTATION_CONTEXT('','3D')
);
#19472=(
LENGTH_UNIT()
NAMED_UNIT(*)
SI_UNIT(.CENTI.,.METRE.)
);
#19474=(
NAMED_UNIT(*)
PLANE_ANGLE_UNIT()
SI_UNIT($,.RADIAN.)
);
#19475=(
NAMED_UNIT(*)
SI_UNIT($,.STERADIAN.)
SOLID_ANGLE_UNIT()
);
#19483=SHAPE_DEFINITION_REPRESENTATION(#19495,#19523);
#19495=PRODUCT_DEFINITION_SHAPE('',$,#19536);
#19523=SHAPE_REPRESENTATION('',(#7525),#19466);
#19528=PRODUCT_DEFINITION_CONTEXT('part definition',#19566,'design');
#19536=PRODUCT_DEFINITION('2026-11-10-01-30-02-390',
'Lower structural shell',#19548,#19528);
#19548=PRODUCT_DEFINITION_FORMATION('',$,#19575);
#19566=APPLICATION_CONTEXT(
'Core Data for Automotive Mechanical Design Process');
#19567=PRODUCT_CONTEXT('part definition',#19566,'mechanical');
#19575=PRODUCT('2026-11-10-01-30-02-390','Lower structural shell',$,(#19567));
#19584=PRESENTATION_STYLE_ASSIGNMENT((#19592));
#19592=SURFACE_STYLE_USAGE(.BOTH.,#19600);
#19600=SURFACE_SIDE_STYLE('',(#19608));
#19608=SURFACE_STYLE_FILL_AREA(#19616);
#19616=FILL_AREA_STYLE('Structural dark blue',(#19624));
#19624=FILL_AREA_STYLE_COLOUR('Structural dark blue',#19632);
#19632=COLOUR_RGB('Structural dark blue',0.0901960784313725,0.270588235294118,
0.513725490196078);
ENDSEC;
END-ISO-10303-21;
